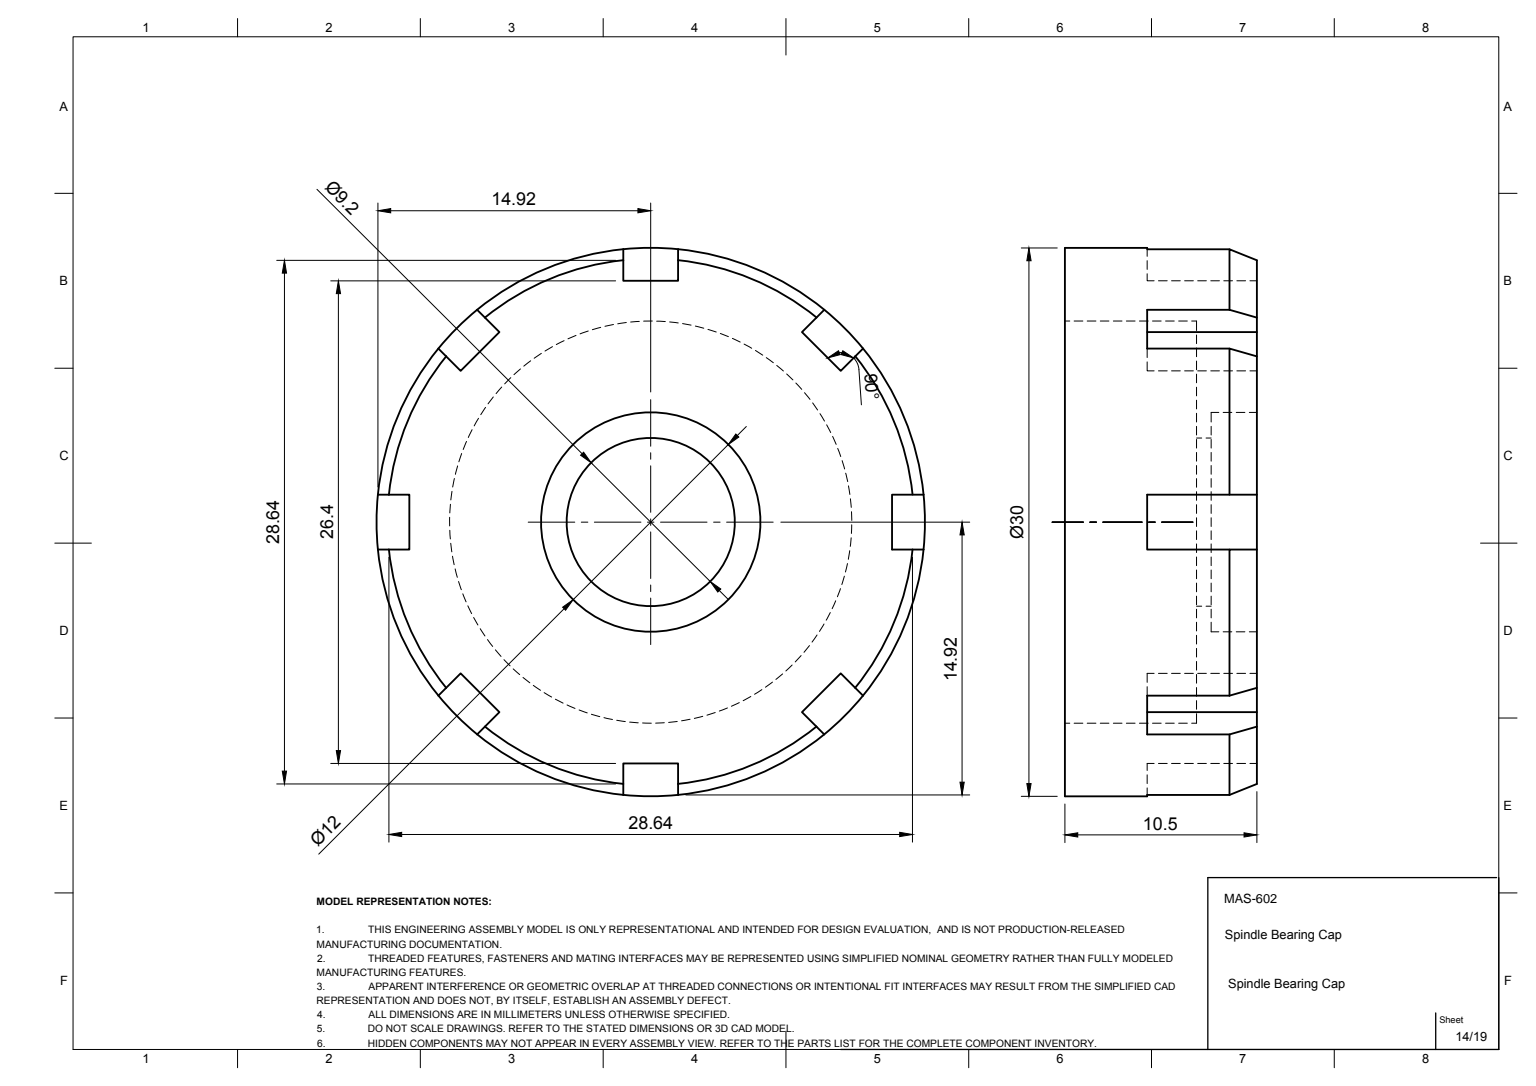
ISO-10303-21;
HEADER;
/* Generated by software containing ST-Developer
 * from STEP Tools, Inc. (www.steptools.com) 
 */

FILE_DESCRIPTION(
/* description */ (''),
/* implementation_level */ '2;1');

FILE_NAME(
/* name */ 'Spindle Bearing Cap.step',
/* time_stamp */ '2026-10-15T14:42:47-07:00',
/* author */ (''),
/* organization */ (''),
/* preprocessor_version */ 'ST-DEVELOPER v20.2',
/* originating_system */ 'Autodesk Translation Framework v15.15.0.0',
/* authorisation */ '');

FILE_SCHEMA (('AUTOMOTIVE_DESIGN { 1 0 10303 214 3 1 1 }'));
ENDSEC;

DATA;
#10=MECHANICAL_DESIGN_GEOMETRIC_PRESENTATION_REPRESENTATION('',(#242),#85789);
#131=(
BOUNDED_CURVE()
B_SPLINE_CURVE(2,(#77398,#77399,#77400),.UNSPECIFIED.,.F.,.F.)
B_SPLINE_CURVE_WITH_KNOTS((3,3),(0.,0.161672183572005),.UNSPECIFIED.)
CURVE()
GEOMETRIC_REPRESENTATION_ITEM()
RATIONAL_B_SPLINE_CURVE((1.,1.00021050527521,1.))
REPRESENTATION_ITEM('')
);
#132=(
BOUNDED_CURVE()
B_SPLINE_CURVE(2,(#77406,#77407,#77408),.UNSPECIFIED.,.F.,.F.)
B_SPLINE_CURVE_WITH_KNOTS((3,3),(0.,0.161672183572005),.UNSPECIFIED.)
CURVE()
GEOMETRIC_REPRESENTATION_ITEM()
RATIONAL_B_SPLINE_CURVE((1.,1.00021050550154,1.))
REPRESENTATION_ITEM('')
);
#133=(
BOUNDED_CURVE()
B_SPLINE_CURVE(2,(#77482,#77483,#77484),.UNSPECIFIED.,.F.,.F.)
B_SPLINE_CURVE_WITH_KNOTS((3,3),(0.,0.161672183572003),.UNSPECIFIED.)
CURVE()
GEOMETRIC_REPRESENTATION_ITEM()
RATIONAL_B_SPLINE_CURVE((1.,1.00021050513902,1.))
REPRESENTATION_ITEM('')
);
#134=(
BOUNDED_CURVE()
B_SPLINE_CURVE(2,(#77487,#77488,#77489),.UNSPECIFIED.,.F.,.F.)
B_SPLINE_CURVE_WITH_KNOTS((3,3),(0.,0.161672183572005),.UNSPECIFIED.)
CURVE()
GEOMETRIC_REPRESENTATION_ITEM()
RATIONAL_B_SPLINE_CURVE((1.,1.00021050510688,1.))
REPRESENTATION_ITEM('')
);
#135=(
BOUNDED_CURVE()
B_SPLINE_CURVE(2,(#77498,#77499,#77500),.UNSPECIFIED.,.F.,.F.)
B_SPLINE_CURVE_WITH_KNOTS((3,3),(0.,0.161672183572005),.UNSPECIFIED.)
CURVE()
GEOMETRIC_REPRESENTATION_ITEM()
RATIONAL_B_SPLINE_CURVE((1.,1.00021050528206,1.))
REPRESENTATION_ITEM('')
);
#136=(
BOUNDED_CURVE()
B_SPLINE_CURVE(2,(#77513,#77514,#77515),.UNSPECIFIED.,.F.,.F.)
B_SPLINE_CURVE_WITH_KNOTS((3,3),(0.,0.161672183572005),.UNSPECIFIED.)
CURVE()
GEOMETRIC_REPRESENTATION_ITEM()
RATIONAL_B_SPLINE_CURVE((1.,1.00021050523753,1.))
REPRESENTATION_ITEM('')
);
#137=(
BOUNDED_CURVE()
B_SPLINE_CURVE(2,(#77524,#77525,#77526),.UNSPECIFIED.,.F.,.F.)
B_SPLINE_CURVE_WITH_KNOTS((3,3),(0.,0.161672183572005),.UNSPECIFIED.)
CURVE()
GEOMETRIC_REPRESENTATION_ITEM()
RATIONAL_B_SPLINE_CURVE((1.,1.00021050533942,1.))
REPRESENTATION_ITEM('')
);
#138=(
BOUNDED_CURVE()
B_SPLINE_CURVE(2,(#77539,#77540,#77541),.UNSPECIFIED.,.F.,.F.)
B_SPLINE_CURVE_WITH_KNOTS((3,3),(0.,0.161672183572005),.UNSPECIFIED.)
CURVE()
GEOMETRIC_REPRESENTATION_ITEM()
RATIONAL_B_SPLINE_CURVE((1.,1.00021050540546,1.))
REPRESENTATION_ITEM('')
);
#139=(
BOUNDED_CURVE()
B_SPLINE_CURVE(2,(#77550,#77551,#77552),.UNSPECIFIED.,.F.,.F.)
B_SPLINE_CURVE_WITH_KNOTS((3,3),(0.,0.161672183572005),.UNSPECIFIED.)
CURVE()
GEOMETRIC_REPRESENTATION_ITEM()
RATIONAL_B_SPLINE_CURVE((1.,1.00021050533233,1.))
REPRESENTATION_ITEM('')
);
#140=(
BOUNDED_CURVE()
B_SPLINE_CURVE(2,(#77567,#77568,#77569),.UNSPECIFIED.,.F.,.F.)
B_SPLINE_CURVE_WITH_KNOTS((3,3),(0.,0.161672183572005),.UNSPECIFIED.)
CURVE()
GEOMETRIC_REPRESENTATION_ITEM()
RATIONAL_B_SPLINE_CURVE((1.,1.00021050531619,1.))
REPRESENTATION_ITEM('')
);
#141=(
BOUNDED_CURVE()
B_SPLINE_CURVE(2,(#77578,#77579,#77580),.UNSPECIFIED.,.F.,.F.)
B_SPLINE_CURVE_WITH_KNOTS((3,3),(0.,0.161672183572005),.UNSPECIFIED.)
CURVE()
GEOMETRIC_REPRESENTATION_ITEM()
RATIONAL_B_SPLINE_CURVE((1.,1.00021050600963,1.))
REPRESENTATION_ITEM('')
);
#142=(
BOUNDED_CURVE()
B_SPLINE_CURVE(2,(#77593,#77594,#77595),.UNSPECIFIED.,.F.,.F.)
B_SPLINE_CURVE_WITH_KNOTS((3,3),(0.,0.161672183572005),.UNSPECIFIED.)
CURVE()
GEOMETRIC_REPRESENTATION_ITEM()
RATIONAL_B_SPLINE_CURVE((1.,1.00021050495933,1.))
REPRESENTATION_ITEM('')
);
#143=(
BOUNDED_CURVE()
B_SPLINE_CURVE(2,(#77604,#77605,#77606),.UNSPECIFIED.,.F.,.F.)
B_SPLINE_CURVE_WITH_KNOTS((3,3),(0.,0.161672183572005),.UNSPECIFIED.)
CURVE()
GEOMETRIC_REPRESENTATION_ITEM()
RATIONAL_B_SPLINE_CURVE((1.,1.00021050494585,1.))
REPRESENTATION_ITEM('')
);
#144=(
BOUNDED_CURVE()
B_SPLINE_CURVE(2,(#77619,#77620,#77621),.UNSPECIFIED.,.F.,.F.)
B_SPLINE_CURVE_WITH_KNOTS((3,3),(0.,0.161672183572003),.UNSPECIFIED.)
CURVE()
GEOMETRIC_REPRESENTATION_ITEM()
RATIONAL_B_SPLINE_CURVE((1.,1.00021050534925,1.))
REPRESENTATION_ITEM('')
);
#145=(
BOUNDED_CURVE()
B_SPLINE_CURVE(2,(#77631,#77632,#77633),.UNSPECIFIED.,.F.,.F.)
B_SPLINE_CURVE_WITH_KNOTS((3,3),(0.,0.161672183572003),.UNSPECIFIED.)
CURVE()
GEOMETRIC_REPRESENTATION_ITEM()
RATIONAL_B_SPLINE_CURVE((1.,1.00021050497678,1.))
REPRESENTATION_ITEM('')
);
#146=(
BOUNDED_CURVE()
B_SPLINE_CURVE(2,(#77645,#77646,#77647),.UNSPECIFIED.,.F.,.F.)
B_SPLINE_CURVE_WITH_KNOTS((3,3),(0.,0.161672183572003),.UNSPECIFIED.)
CURVE()
GEOMETRIC_REPRESENTATION_ITEM()
RATIONAL_B_SPLINE_CURVE((1.,1.00021050515309,1.))
REPRESENTATION_ITEM('')
);
#169=CONICAL_SURFACE('',#10614,1.47,0.380506377112364);
#170=CONICAL_SURFACE('',#10616,1.47,0.380506377112364);
#171=CONICAL_SURFACE('',#10623,1.47,0.380506377112364);
#172=CONICAL_SURFACE('',#10630,1.47,0.380506377112364);
#173=CONICAL_SURFACE('',#10638,1.47,0.380506377112364);
#174=CONICAL_SURFACE('',#10645,1.47,0.380506377112364);
#175=CONICAL_SURFACE('',#10652,1.47,0.380506377112364);
#176=CONICAL_SURFACE('',#10659,1.47,0.380506377112364);
#206=SHAPE_REPRESENTATION_RELATIONSHIP('SRR','None',#85871,#224);
#224=ADVANCED_BREP_SHAPE_REPRESENTATION('',(#260),#85779);
#242=STYLED_ITEM('',(#85970),#260);
#260=MANIFOLD_SOLID_BREP('Body1',#9889);
#455=FACE_BOUND('',#3306,.T.);
#456=FACE_BOUND('',#3345,.T.);
#457=FACE_BOUND('',#3348,.T.);
#458=FACE_BOUND('',#3352,.T.);
#1118=PLANE('',#10599);
#1119=PLANE('',#10600);
#1120=PLANE('',#10601);
#1121=PLANE('',#10602);
#1122=PLANE('',#10604);
#1123=PLANE('',#10618);
#1124=PLANE('',#10619);
#1125=PLANE('',#10620);
#1126=PLANE('',#10621);
#1127=PLANE('',#10625);
#1128=PLANE('',#10626);
#1129=PLANE('',#10627);
#1130=PLANE('',#10628);
#1131=PLANE('',#10632);
#1132=PLANE('',#10633);
#1133=PLANE('',#10634);
#1134=PLANE('',#10635);
#1135=PLANE('',#10640);
#1136=PLANE('',#10641);
#1137=PLANE('',#10642);
#1138=PLANE('',#10643);
#1139=PLANE('',#10647);
#1140=PLANE('',#10648);
#1141=PLANE('',#10649);
#1142=PLANE('',#10650);
#1143=PLANE('',#10654);
#1144=PLANE('',#10655);
#1145=PLANE('',#10656);
#1146=PLANE('',#10657);
#1147=PLANE('',#10661);
#1148=PLANE('',#10662);
#1149=PLANE('',#10663);
#1150=PLANE('',#10664);
#1151=PLANE('',#10669);
#1152=PLANE('',#10673);
#1153=PLANE('',#10678);
#1539=LINE('',#77391,#2075);
#1540=LINE('',#77393,#2076);
#1541=LINE('',#77395,#2077);
#1542=LINE('',#77397,#2078);
#1543=LINE('',#77404,#2079);
#1544=LINE('',#77410,#2080);
#1545=LINE('',#77412,#2081);
#1546=LINE('',#77413,#2082);
#1547=LINE('',#77415,#2083);
#1548=LINE('',#77416,#2084);
#1549=LINE('',#77423,#2085);
#1550=LINE('',#77425,#2086);
#1551=LINE('',#77427,#2087);
#1552=LINE('',#77431,#2088);
#1553=LINE('',#77433,#2089);
#1554=LINE('',#77435,#2090);
#1555=LINE('',#77439,#2091);
#1556=LINE('',#77441,#2092);
#1557=LINE('',#77443,#2093);
#1558=LINE('',#77447,#2094);
#1559=LINE('',#77449,#2095);
#1560=LINE('',#77451,#2096);
#1561=LINE('',#77455,#2097);
#1562=LINE('',#77457,#2098);
#1563=LINE('',#77459,#2099);
#1564=LINE('',#77463,#2100);
#1565=LINE('',#77465,#2101);
#1566=LINE('',#77467,#2102);
#1567=LINE('',#77471,#2103);
#1568=LINE('',#77473,#2104);
#1569=LINE('',#77475,#2105);
#1570=LINE('',#77494,#2106);
#1571=LINE('',#77496,#2107);
#1572=LINE('',#77497,#2108);
#1573=LINE('',#77503,#2109);
#1574=LINE('',#77505,#2110);
#1575=LINE('',#77506,#2111);
#1576=LINE('',#77508,#2112);
#1577=LINE('',#77520,#2113);
#1578=LINE('',#77522,#2114);
#1579=LINE('',#77523,#2115);
#1580=LINE('',#77529,#2116);
#1581=LINE('',#77531,#2117);
#1582=LINE('',#77532,#2118);
#1583=LINE('',#77534,#2119);
#1584=LINE('',#77546,#2120);
#1585=LINE('',#77548,#2121);
#1586=LINE('',#77549,#2122);
#1587=LINE('',#77555,#2123);
#1588=LINE('',#77557,#2124);
#1589=LINE('',#77558,#2125);
#1590=LINE('',#77560,#2126);
#1591=LINE('',#77574,#2127);
#1592=LINE('',#77576,#2128);
#1593=LINE('',#77577,#2129);
#1594=LINE('',#77583,#2130);
#1595=LINE('',#77585,#2131);
#1596=LINE('',#77586,#2132);
#1597=LINE('',#77588,#2133);
#1598=LINE('',#77600,#2134);
#1599=LINE('',#77602,#2135);
#1600=LINE('',#77603,#2136);
#1601=LINE('',#77609,#2137);
#1602=LINE('',#77611,#2138);
#1603=LINE('',#77612,#2139);
#1604=LINE('',#77614,#2140);
#1605=LINE('',#77625,#2141);
#1606=LINE('',#77627,#2142);
#1607=LINE('',#77628,#2143);
#1608=LINE('',#77635,#2144);
#1609=LINE('',#77637,#2145);
#1610=LINE('',#77638,#2146);
#1611=LINE('',#77640,#2147);
#1612=LINE('',#77651,#2148);
#1613=LINE('',#77653,#2149);
#1614=LINE('',#77654,#2150);
#1615=LINE('',#77657,#2151);
#1616=LINE('',#77659,#2152);
#1617=LINE('',#77660,#2153);
#1618=LINE('',#77662,#2154);
#1619=LINE('',#77669,#2155);
#1620=LINE('',#77676,#2156);
#1621=LINE('',#77682,#2157);
#1622=LINE('',#77686,#2158);
#2075=VECTOR('',#12303,1.);
#2076=VECTOR('',#12304,1.);
#2077=VECTOR('',#12305,1.);
#2078=VECTOR('',#12306,1.);
#2079=VECTOR('',#12309,1.);
#2080=VECTOR('',#12310,1.);
#2081=VECTOR('',#12311,1.);
#2082=VECTOR('',#12312,1.);
#2083=VECTOR('',#12315,1.);
#2084=VECTOR('',#12316,1.);
#2085=VECTOR('',#12325,1.);
#2086=VECTOR('',#12326,1.);
#2087=VECTOR('',#12327,1.);
#2088=VECTOR('',#12330,1.);
#2089=VECTOR('',#12331,1.);
#2090=VECTOR('',#12332,1.);
#2091=VECTOR('',#12335,1.);
#2092=VECTOR('',#12336,1.);
#2093=VECTOR('',#12337,1.);
#2094=VECTOR('',#12340,1.);
#2095=VECTOR('',#12341,1.);
#2096=VECTOR('',#12342,1.);
#2097=VECTOR('',#12345,1.);
#2098=VECTOR('',#12346,1.);
#2099=VECTOR('',#12347,1.);
#2100=VECTOR('',#12350,1.);
#2101=VECTOR('',#12351,1.);
#2102=VECTOR('',#12352,1.);
#2103=VECTOR('',#12355,1.);
#2104=VECTOR('',#12356,1.);
#2105=VECTOR('',#12357,1.);
#2106=VECTOR('',#12372,1.);
#2107=VECTOR('',#12373,1.);
#2108=VECTOR('',#12374,1.);
#2109=VECTOR('',#12377,1.);
#2110=VECTOR('',#12378,1.);
#2111=VECTOR('',#12379,1.);
#2112=VECTOR('',#12382,1.);
#2113=VECTOR('',#12393,1.);
#2114=VECTOR('',#12394,1.);
#2115=VECTOR('',#12395,1.);
#2116=VECTOR('',#12398,1.);
#2117=VECTOR('',#12399,1.);
#2118=VECTOR('',#12400,1.);
#2119=VECTOR('',#12403,1.);
#2120=VECTOR('',#12414,1.);
#2121=VECTOR('',#12415,1.);
#2122=VECTOR('',#12416,1.);
#2123=VECTOR('',#12419,1.);
#2124=VECTOR('',#12420,1.);
#2125=VECTOR('',#12421,1.);
#2126=VECTOR('',#12424,1.);
#2127=VECTOR('',#12437,1.);
#2128=VECTOR('',#12438,1.);
#2129=VECTOR('',#12439,1.);
#2130=VECTOR('',#12442,1.);
#2131=VECTOR('',#12443,1.);
#2132=VECTOR('',#12444,1.);
#2133=VECTOR('',#12447,1.);
#2134=VECTOR('',#12458,1.);
#2135=VECTOR('',#12459,1.);
#2136=VECTOR('',#12460,1.);
#2137=VECTOR('',#12463,1.);
#2138=VECTOR('',#12464,1.);
#2139=VECTOR('',#12465,1.);
#2140=VECTOR('',#12468,1.);
#2141=VECTOR('',#12479,1.);
#2142=VECTOR('',#12480,1.);
#2143=VECTOR('',#12481,1.);
#2144=VECTOR('',#12484,1.);
#2145=VECTOR('',#12485,1.);
#2146=VECTOR('',#12486,1.);
#2147=VECTOR('',#12489,1.);
#2148=VECTOR('',#12500,1.);
#2149=VECTOR('',#12501,1.);
#2150=VECTOR('',#12502,1.);
#2151=VECTOR('',#12505,1.);
#2152=VECTOR('',#12506,1.);
#2153=VECTOR('',#12507,1.);
#2154=VECTOR('',#12510,1.);
#2155=VECTOR('',#12519,1.1);
#2156=VECTOR('',#12528,0.46);
#2157=VECTOR('',#12537,1.5);
#2158=VECTOR('',#12542,0.6);
#2344=CYLINDRICAL_SURFACE('',#10666,1.1);
#2345=CYLINDRICAL_SURFACE('',#10671,0.46);
#2346=CYLINDRICAL_SURFACE('',#10675,1.5);
#2347=CYLINDRICAL_SURFACE('',#10676,0.6);
#2731=FACE_OUTER_BOUND('',#3301,.T.);
#2732=FACE_OUTER_BOUND('',#3302,.T.);
#2733=FACE_OUTER_BOUND('',#3303,.T.);
#2734=FACE_OUTER_BOUND('',#3304,.T.);
#2735=FACE_OUTER_BOUND('',#3305,.T.);
#2736=FACE_OUTER_BOUND('',#3307,.T.);
#2737=FACE_OUTER_BOUND('',#3308,.T.);
#2738=FACE_OUTER_BOUND('',#3309,.T.);
#2739=FACE_OUTER_BOUND('',#3310,.T.);
#2740=FACE_OUTER_BOUND('',#3311,.T.);
#2741=FACE_OUTER_BOUND('',#3312,.T.);
#2742=FACE_OUTER_BOUND('',#3313,.T.);
#2743=FACE_OUTER_BOUND('',#3314,.T.);
#2744=FACE_OUTER_BOUND('',#3315,.T.);
#2745=FACE_OUTER_BOUND('',#3316,.T.);
#2746=FACE_OUTER_BOUND('',#3317,.T.);
#2747=FACE_OUTER_BOUND('',#3318,.T.);
#2748=FACE_OUTER_BOUND('',#3319,.T.);
#2749=FACE_OUTER_BOUND('',#3320,.T.);
#2750=FACE_OUTER_BOUND('',#3321,.T.);
#2751=FACE_OUTER_BOUND('',#3322,.T.);
#2752=FACE_OUTER_BOUND('',#3323,.T.);
#2753=FACE_OUTER_BOUND('',#3324,.T.);
#2754=FACE_OUTER_BOUND('',#3325,.T.);
#2755=FACE_OUTER_BOUND('',#3326,.T.);
#2756=FACE_OUTER_BOUND('',#3327,.T.);
#2757=FACE_OUTER_BOUND('',#3328,.T.);
#2758=FACE_OUTER_BOUND('',#3329,.T.);
#2759=FACE_OUTER_BOUND('',#3330,.T.);
#2760=FACE_OUTER_BOUND('',#3331,.T.);
#2761=FACE_OUTER_BOUND('',#3332,.T.);
#2762=FACE_OUTER_BOUND('',#3333,.T.);
#2763=FACE_OUTER_BOUND('',#3334,.T.);
#2764=FACE_OUTER_BOUND('',#3335,.T.);
#2765=FACE_OUTER_BOUND('',#3336,.T.);
#2766=FACE_OUTER_BOUND('',#3337,.T.);
#2767=FACE_OUTER_BOUND('',#3338,.T.);
#2768=FACE_OUTER_BOUND('',#3339,.T.);
#2769=FACE_OUTER_BOUND('',#3340,.T.);
#2770=FACE_OUTER_BOUND('',#3341,.T.);
#2771=FACE_OUTER_BOUND('',#3342,.T.);
#2772=FACE_OUTER_BOUND('',#3343,.T.);
#2773=FACE_OUTER_BOUND('',#3344,.T.);
#2774=FACE_OUTER_BOUND('',#3346,.T.);
#2775=FACE_OUTER_BOUND('',#3347,.T.);
#2776=FACE_OUTER_BOUND('',#3349,.T.);
#2777=FACE_OUTER_BOUND('',#3350,.T.);
#2778=FACE_OUTER_BOUND('',#3351,.T.);
#3301=EDGE_LOOP('',(#8463,#8464,#8465,#8466,#8467));
#3302=EDGE_LOOP('',(#8468,#8469,#8470,#8471,#8472));
#3303=EDGE_LOOP('',(#8473,#8474,#8475,#8476));
#3304=EDGE_LOOP('',(#8477,#8478,#8479,#8480));
#3305=EDGE_LOOP('',(#8481,#8482,#8483,#8484,#8485,#8486,#8487,#8488,#8489,
#8490,#8491,#8492,#8493,#8494,#8495,#8496,#8497,#8498,#8499,#8500,#8501,
#8502,#8503,#8504,#8505,#8506,#8507,#8508,#8509,#8510,#8511,#8512));
#3306=EDGE_LOOP('',(#8513));
#3307=EDGE_LOOP('',(#8514,#8515,#8516,#8517));
#3308=EDGE_LOOP('',(#8518,#8519,#8520,#8521));
#3309=EDGE_LOOP('',(#8522,#8523,#8524,#8525,#8526));
#3310=EDGE_LOOP('',(#8527,#8528,#8529,#8530,#8531));
#3311=EDGE_LOOP('',(#8532,#8533,#8534,#8535));
#3312=EDGE_LOOP('',(#8536,#8537,#8538,#8539));
#3313=EDGE_LOOP('',(#8540,#8541,#8542,#8543));
#3314=EDGE_LOOP('',(#8544,#8545,#8546,#8547,#8548));
#3315=EDGE_LOOP('',(#8549,#8550,#8551,#8552,#8553));
#3316=EDGE_LOOP('',(#8554,#8555,#8556,#8557));
#3317=EDGE_LOOP('',(#8558,#8559,#8560,#8561));
#3318=EDGE_LOOP('',(#8562,#8563,#8564,#8565));
#3319=EDGE_LOOP('',(#8566,#8567,#8568,#8569,#8570));
#3320=EDGE_LOOP('',(#8571,#8572,#8573,#8574,#8575));
#3321=EDGE_LOOP('',(#8576,#8577,#8578,#8579));
#3322=EDGE_LOOP('',(#8580,#8581,#8582,#8583,#8584));
#3323=EDGE_LOOP('',(#8585,#8586,#8587,#8588));
#3324=EDGE_LOOP('',(#8589,#8590,#8591,#8592,#8593));
#3325=EDGE_LOOP('',(#8594,#8595,#8596,#8597,#8598));
#3326=EDGE_LOOP('',(#8599,#8600,#8601,#8602));
#3327=EDGE_LOOP('',(#8603,#8604,#8605,#8606));
#3328=EDGE_LOOP('',(#8607,#8608,#8609,#8610));
#3329=EDGE_LOOP('',(#8611,#8612,#8613,#8614,#8615));
#3330=EDGE_LOOP('',(#8616,#8617,#8618,#8619,#8620));
#3331=EDGE_LOOP('',(#8621,#8622,#8623,#8624));
#3332=EDGE_LOOP('',(#8625,#8626,#8627,#8628));
#3333=EDGE_LOOP('',(#8629,#8630,#8631,#8632));
#3334=EDGE_LOOP('',(#8633,#8634,#8635,#8636,#8637));
#3335=EDGE_LOOP('',(#8638,#8639,#8640,#8641,#8642));
#3336=EDGE_LOOP('',(#8643,#8644,#8645,#8646));
#3337=EDGE_LOOP('',(#8647,#8648,#8649,#8650));
#3338=EDGE_LOOP('',(#8651,#8652,#8653,#8654));
#3339=EDGE_LOOP('',(#8655,#8656,#8657,#8658,#8659));
#3340=EDGE_LOOP('',(#8660,#8661,#8662,#8663,#8664));
#3341=EDGE_LOOP('',(#8665,#8666,#8667,#8668));
#3342=EDGE_LOOP('',(#8669,#8670,#8671,#8672));
#3343=EDGE_LOOP('',(#8673,#8674,#8675,#8676));
#3344=EDGE_LOOP('',(#8677));
#3345=EDGE_LOOP('',(#8678));
#3346=EDGE_LOOP('',(#8679,#8680,#8681,#8682));
#3347=EDGE_LOOP('',(#8683));
#3348=EDGE_LOOP('',(#8684));
#3349=EDGE_LOOP('',(#8685,#8686,#8687,#8688,#8689,#8690,#8691,#8692,#8693,
#8694,#8695,#8696,#8697,#8698,#8699,#8700,#8701,#8702,#8703,#8704,#8705,
#8706,#8707,#8708,#8709,#8710,#8711,#8712,#8713,#8714,#8715,#8716,#8717,
#8718,#8719,#8720));
#3350=EDGE_LOOP('',(#8721,#8722,#8723,#8724));
#3351=EDGE_LOOP('',(#8725));
#3352=EDGE_LOOP('',(#8726));
#3744=CIRCLE('',#10603,1.5);
#3745=CIRCLE('',#10605,1.44);
#3746=CIRCLE('',#10606,1.44);
#3747=CIRCLE('',#10607,1.44);
#3748=CIRCLE('',#10608,1.44);
#3749=CIRCLE('',#10609,1.44);
#3750=CIRCLE('',#10610,1.44);
#3751=CIRCLE('',#10611,1.44);
#3752=CIRCLE('',#10612,1.44);
#3753=CIRCLE('',#10613,0.6);
#3754=CIRCLE('',#10615,1.5);
#3755=CIRCLE('',#10617,1.5);
#3756=CIRCLE('',#10622,1.5);
#3757=CIRCLE('',#10624,1.5);
#3758=CIRCLE('',#10629,1.5);
#3759=CIRCLE('',#10631,1.5);
#3760=CIRCLE('',#10636,1.5);
#3761=CIRCLE('',#10637,1.5);
#3762=CIRCLE('',#10639,1.5);
#3763=CIRCLE('',#10644,1.5);
#3764=CIRCLE('',#10646,1.5);
#3765=CIRCLE('',#10651,1.5);
#3766=CIRCLE('',#10653,1.5);
#3767=CIRCLE('',#10658,1.5);
#3768=CIRCLE('',#10660,1.5);
#3769=CIRCLE('',#10665,1.5);
#3770=CIRCLE('',#10667,1.1);
#3771=CIRCLE('',#10668,1.1);
#3772=CIRCLE('',#10670,0.46);
#3773=CIRCLE('',#10672,0.46);
#3774=CIRCLE('',#10674,1.5);
#3775=CIRCLE('',#10677,0.6);
#4619=VERTEX_POINT('',#77389);
#4620=VERTEX_POINT('',#77390);
#4621=VERTEX_POINT('',#77392);
#4622=VERTEX_POINT('',#77394);
#4623=VERTEX_POINT('',#77396);
#4624=VERTEX_POINT('',#77402);
#4625=VERTEX_POINT('',#77403);
#4626=VERTEX_POINT('',#77405);
#4627=VERTEX_POINT('',#77409);
#4628=VERTEX_POINT('',#77411);
#4629=VERTEX_POINT('',#77420);
#4630=VERTEX_POINT('',#77422);
#4631=VERTEX_POINT('',#77424);
#4632=VERTEX_POINT('',#77426);
#4633=VERTEX_POINT('',#77428);
#4634=VERTEX_POINT('',#77430);
#4635=VERTEX_POINT('',#77432);
#4636=VERTEX_POINT('',#77434);
#4637=VERTEX_POINT('',#77436);
#4638=VERTEX_POINT('',#77438);
#4639=VERTEX_POINT('',#77440);
#4640=VERTEX_POINT('',#77442);
#4641=VERTEX_POINT('',#77444);
#4642=VERTEX_POINT('',#77446);
#4643=VERTEX_POINT('',#77448);
#4644=VERTEX_POINT('',#77450);
#4645=VERTEX_POINT('',#77452);
#4646=VERTEX_POINT('',#77454);
#4647=VERTEX_POINT('',#77456);
#4648=VERTEX_POINT('',#77458);
#4649=VERTEX_POINT('',#77460);
#4650=VERTEX_POINT('',#77462);
#4651=VERTEX_POINT('',#77464);
#4652=VERTEX_POINT('',#77466);
#4653=VERTEX_POINT('',#77468);
#4654=VERTEX_POINT('',#77470);
#4655=VERTEX_POINT('',#77472);
#4656=VERTEX_POINT('',#77474);
#4657=VERTEX_POINT('',#77477);
#4658=VERTEX_POINT('',#77480);
#4659=VERTEX_POINT('',#77486);
#4660=VERTEX_POINT('',#77492);
#4661=VERTEX_POINT('',#77493);
#4662=VERTEX_POINT('',#77495);
#4663=VERTEX_POINT('',#77502);
#4664=VERTEX_POINT('',#77504);
#4665=VERTEX_POINT('',#77512);
#4666=VERTEX_POINT('',#77518);
#4667=VERTEX_POINT('',#77519);
#4668=VERTEX_POINT('',#77521);
#4669=VERTEX_POINT('',#77528);
#4670=VERTEX_POINT('',#77530);
#4671=VERTEX_POINT('',#77538);
#4672=VERTEX_POINT('',#77544);
#4673=VERTEX_POINT('',#77545);
#4674=VERTEX_POINT('',#77547);
#4675=VERTEX_POINT('',#77554);
#4676=VERTEX_POINT('',#77556);
#4677=VERTEX_POINT('',#77562);
#4678=VERTEX_POINT('',#77566);
#4679=VERTEX_POINT('',#77572);
#4680=VERTEX_POINT('',#77573);
#4681=VERTEX_POINT('',#77575);
#4682=VERTEX_POINT('',#77582);
#4683=VERTEX_POINT('',#77584);
#4684=VERTEX_POINT('',#77592);
#4685=VERTEX_POINT('',#77598);
#4686=VERTEX_POINT('',#77599);
#4687=VERTEX_POINT('',#77601);
#4688=VERTEX_POINT('',#77608);
#4689=VERTEX_POINT('',#77610);
#4690=VERTEX_POINT('',#77618);
#4691=VERTEX_POINT('',#77624);
#4692=VERTEX_POINT('',#77626);
#4693=VERTEX_POINT('',#77630);
#4694=VERTEX_POINT('',#77634);
#4695=VERTEX_POINT('',#77636);
#4696=VERTEX_POINT('',#77644);
#4697=VERTEX_POINT('',#77650);
#4698=VERTEX_POINT('',#77652);
#4699=VERTEX_POINT('',#77656);
#4700=VERTEX_POINT('',#77658);
#4701=VERTEX_POINT('',#77666);
#4702=VERTEX_POINT('',#77668);
#4703=VERTEX_POINT('',#77672);
#4704=VERTEX_POINT('',#77675);
#4705=VERTEX_POINT('',#77679);
#4706=VERTEX_POINT('',#77684);
#5959=EDGE_CURVE('',#4619,#4620,#1539,.T.);
#5960=EDGE_CURVE('',#4619,#4621,#1540,.T.);
#5961=EDGE_CURVE('',#4622,#4621,#1541,.T.);
#5962=EDGE_CURVE('',#4623,#4622,#1542,.T.);
#5963=EDGE_CURVE('',#4620,#4623,#131,.T.);
#5964=EDGE_CURVE('',#4624,#4625,#1543,.T.);
#5965=EDGE_CURVE('',#4626,#4624,#132,.T.);
#5966=EDGE_CURVE('',#4627,#4626,#1544,.T.);
#5967=EDGE_CURVE('',#4627,#4628,#1545,.T.);
#5968=EDGE_CURVE('',#4628,#4625,#1546,.T.);
#5969=EDGE_CURVE('',#4622,#4627,#1547,.T.);
#5970=EDGE_CURVE('',#4621,#4628,#1548,.T.);
#5971=EDGE_CURVE('',#4625,#4619,#3744,.T.);
#5972=EDGE_CURVE('',#4626,#4629,#3745,.T.);
#5973=EDGE_CURVE('',#4629,#4630,#1549,.T.);
#5974=EDGE_CURVE('',#4630,#4631,#1550,.T.);
#5975=EDGE_CURVE('',#4631,#4632,#1551,.T.);
#5976=EDGE_CURVE('',#4632,#4633,#3746,.T.);
#5977=EDGE_CURVE('',#4633,#4634,#1552,.T.);
#5978=EDGE_CURVE('',#4634,#4635,#1553,.T.);
#5979=EDGE_CURVE('',#4635,#4636,#1554,.T.);
#5980=EDGE_CURVE('',#4636,#4637,#3747,.T.);
#5981=EDGE_CURVE('',#4637,#4638,#1555,.T.);
#5982=EDGE_CURVE('',#4638,#4639,#1556,.T.);
#5983=EDGE_CURVE('',#4639,#4640,#1557,.T.);
#5984=EDGE_CURVE('',#4640,#4641,#3748,.T.);
#5985=EDGE_CURVE('',#4641,#4642,#1558,.T.);
#5986=EDGE_CURVE('',#4642,#4643,#1559,.T.);
#5987=EDGE_CURVE('',#4643,#4644,#1560,.T.);
#5988=EDGE_CURVE('',#4644,#4645,#3749,.T.);
#5989=EDGE_CURVE('',#4645,#4646,#1561,.T.);
#5990=EDGE_CURVE('',#4646,#4647,#1562,.T.);
#5991=EDGE_CURVE('',#4647,#4648,#1563,.T.);
#5992=EDGE_CURVE('',#4648,#4649,#3750,.T.);
#5993=EDGE_CURVE('',#4649,#4650,#1564,.T.);
#5994=EDGE_CURVE('',#4650,#4651,#1565,.T.);
#5995=EDGE_CURVE('',#4651,#4652,#1566,.T.);
#5996=EDGE_CURVE('',#4652,#4653,#3751,.T.);
#5997=EDGE_CURVE('',#4653,#4654,#1567,.T.);
#5998=EDGE_CURVE('',#4654,#4655,#1568,.T.);
#5999=EDGE_CURVE('',#4655,#4656,#1569,.T.);
#6000=EDGE_CURVE('',#4656,#4623,#3752,.T.);
#6001=EDGE_CURVE('',#4657,#4657,#3753,.T.);
#6002=EDGE_CURVE('',#4624,#4658,#3754,.T.);
#6003=EDGE_CURVE('',#4658,#4629,#133,.T.);
#6004=EDGE_CURVE('',#4656,#4659,#134,.T.);
#6005=EDGE_CURVE('',#4659,#4620,#3755,.T.);
#6006=EDGE_CURVE('',#4660,#4661,#1570,.T.);
#6007=EDGE_CURVE('',#4660,#4662,#1571,.T.);
#6008=EDGE_CURVE('',#4654,#4662,#1572,.T.);
#6009=EDGE_CURVE('',#4661,#4653,#135,.T.);
#6010=EDGE_CURVE('',#4659,#4663,#1573,.T.);
#6011=EDGE_CURVE('',#4655,#4664,#1574,.T.);
#6012=EDGE_CURVE('',#4664,#4663,#1575,.T.);
#6013=EDGE_CURVE('',#4662,#4664,#1576,.T.);
#6014=EDGE_CURVE('',#4663,#4660,#3756,.T.);
#6015=EDGE_CURVE('',#4652,#4665,#136,.T.);
#6016=EDGE_CURVE('',#4665,#4661,#3757,.T.);
#6017=EDGE_CURVE('',#4666,#4667,#1577,.T.);
#6018=EDGE_CURVE('',#4666,#4668,#1578,.T.);
#6019=EDGE_CURVE('',#4650,#4668,#1579,.T.);
#6020=EDGE_CURVE('',#4667,#4649,#137,.T.);
#6021=EDGE_CURVE('',#4665,#4669,#1580,.T.);
#6022=EDGE_CURVE('',#4651,#4670,#1581,.T.);
#6023=EDGE_CURVE('',#4670,#4669,#1582,.T.);
#6024=EDGE_CURVE('',#4668,#4670,#1583,.T.);
#6025=EDGE_CURVE('',#4669,#4666,#3758,.T.);
#6026=EDGE_CURVE('',#4648,#4671,#138,.T.);
#6027=EDGE_CURVE('',#4671,#4667,#3759,.T.);
#6028=EDGE_CURVE('',#4672,#4673,#1584,.T.);
#6029=EDGE_CURVE('',#4672,#4674,#1585,.T.);
#6030=EDGE_CURVE('',#4646,#4674,#1586,.T.);
#6031=EDGE_CURVE('',#4673,#4645,#139,.T.);
#6032=EDGE_CURVE('',#4671,#4675,#1587,.T.);
#6033=EDGE_CURVE('',#4647,#4676,#1588,.T.);
#6034=EDGE_CURVE('',#4676,#4675,#1589,.T.);
#6035=EDGE_CURVE('',#4674,#4676,#1590,.T.);
#6036=EDGE_CURVE('',#4675,#4677,#3760,.T.);
#6037=EDGE_CURVE('',#4677,#4672,#3761,.T.);
#6038=EDGE_CURVE('',#4644,#4678,#140,.T.);
#6039=EDGE_CURVE('',#4678,#4673,#3762,.T.);
#6040=EDGE_CURVE('',#4679,#4680,#1591,.T.);
#6041=EDGE_CURVE('',#4679,#4681,#1592,.T.);
#6042=EDGE_CURVE('',#4642,#4681,#1593,.T.);
#6043=EDGE_CURVE('',#4680,#4641,#141,.T.);
#6044=EDGE_CURVE('',#4678,#4682,#1594,.T.);
#6045=EDGE_CURVE('',#4643,#4683,#1595,.T.);
#6046=EDGE_CURVE('',#4683,#4682,#1596,.T.);
#6047=EDGE_CURVE('',#4681,#4683,#1597,.T.);
#6048=EDGE_CURVE('',#4682,#4679,#3763,.T.);
#6049=EDGE_CURVE('',#4640,#4684,#142,.T.);
#6050=EDGE_CURVE('',#4684,#4680,#3764,.T.);
#6051=EDGE_CURVE('',#4685,#4686,#1598,.T.);
#6052=EDGE_CURVE('',#4685,#4687,#1599,.T.);
#6053=EDGE_CURVE('',#4638,#4687,#1600,.T.);
#6054=EDGE_CURVE('',#4686,#4637,#143,.T.);
#6055=EDGE_CURVE('',#4684,#4688,#1601,.T.);
#6056=EDGE_CURVE('',#4639,#4689,#1602,.T.);
#6057=EDGE_CURVE('',#4689,#4688,#1603,.T.);
#6058=EDGE_CURVE('',#4687,#4689,#1604,.T.);
#6059=EDGE_CURVE('',#4688,#4685,#3765,.T.);
#6060=EDGE_CURVE('',#4636,#4690,#144,.T.);
#6061=EDGE_CURVE('',#4690,#4686,#3766,.T.);
#6062=EDGE_CURVE('',#4635,#4691,#1605,.T.);
#6063=EDGE_CURVE('',#4691,#4692,#1606,.T.);
#6064=EDGE_CURVE('',#4690,#4692,#1607,.T.);
#6065=EDGE_CURVE('',#4693,#4633,#145,.T.);
#6066=EDGE_CURVE('',#4694,#4693,#1608,.T.);
#6067=EDGE_CURVE('',#4694,#4695,#1609,.T.);
#6068=EDGE_CURVE('',#4634,#4695,#1610,.T.);
#6069=EDGE_CURVE('',#4695,#4691,#1611,.T.);
#6070=EDGE_CURVE('',#4692,#4694,#3767,.T.);
#6071=EDGE_CURVE('',#4632,#4696,#146,.T.);
#6072=EDGE_CURVE('',#4696,#4693,#3768,.T.);
#6073=EDGE_CURVE('',#4631,#4697,#1612,.T.);
#6074=EDGE_CURVE('',#4697,#4698,#1613,.T.);
#6075=EDGE_CURVE('',#4696,#4698,#1614,.T.);
#6076=EDGE_CURVE('',#4699,#4658,#1615,.T.);
#6077=EDGE_CURVE('',#4699,#4700,#1616,.T.);
#6078=EDGE_CURVE('',#4630,#4700,#1617,.T.);
#6079=EDGE_CURVE('',#4700,#4697,#1618,.T.);
#6080=EDGE_CURVE('',#4698,#4699,#3769,.T.);
#6081=EDGE_CURVE('',#4701,#4701,#3770,.T.);
#6082=EDGE_CURVE('',#4701,#4702,#1619,.T.);
#6083=EDGE_CURVE('',#4702,#4702,#3771,.T.);
#6084=EDGE_CURVE('',#4703,#4703,#3772,.T.);
#6085=EDGE_CURVE('',#4703,#4704,#1620,.T.);
#6086=EDGE_CURVE('',#4704,#4704,#3773,.T.);
#6087=EDGE_CURVE('',#4705,#4705,#3774,.T.);
#6088=EDGE_CURVE('',#4677,#4705,#1621,.T.);
#6089=EDGE_CURVE('',#4706,#4706,#3775,.T.);
#6090=EDGE_CURVE('',#4706,#4657,#1622,.T.);
#8463=ORIENTED_EDGE('',*,*,#5959,.F.);
#8464=ORIENTED_EDGE('',*,*,#5960,.T.);
#8465=ORIENTED_EDGE('',*,*,#5961,.F.);
#8466=ORIENTED_EDGE('',*,*,#5962,.F.);
#8467=ORIENTED_EDGE('',*,*,#5963,.F.);
#8468=ORIENTED_EDGE('',*,*,#5964,.F.);
#8469=ORIENTED_EDGE('',*,*,#5965,.F.);
#8470=ORIENTED_EDGE('',*,*,#5966,.F.);
#8471=ORIENTED_EDGE('',*,*,#5967,.T.);
#8472=ORIENTED_EDGE('',*,*,#5968,.T.);
#8473=ORIENTED_EDGE('',*,*,#5969,.F.);
#8474=ORIENTED_EDGE('',*,*,#5961,.T.);
#8475=ORIENTED_EDGE('',*,*,#5970,.T.);
#8476=ORIENTED_EDGE('',*,*,#5967,.F.);
#8477=ORIENTED_EDGE('',*,*,#5971,.F.);
#8478=ORIENTED_EDGE('',*,*,#5968,.F.);
#8479=ORIENTED_EDGE('',*,*,#5970,.F.);
#8480=ORIENTED_EDGE('',*,*,#5960,.F.);
#8481=ORIENTED_EDGE('',*,*,#5962,.T.);
#8482=ORIENTED_EDGE('',*,*,#5969,.T.);
#8483=ORIENTED_EDGE('',*,*,#5966,.T.);
#8484=ORIENTED_EDGE('',*,*,#5972,.T.);
#8485=ORIENTED_EDGE('',*,*,#5973,.T.);
#8486=ORIENTED_EDGE('',*,*,#5974,.T.);
#8487=ORIENTED_EDGE('',*,*,#5975,.T.);
#8488=ORIENTED_EDGE('',*,*,#5976,.T.);
#8489=ORIENTED_EDGE('',*,*,#5977,.T.);
#8490=ORIENTED_EDGE('',*,*,#5978,.T.);
#8491=ORIENTED_EDGE('',*,*,#5979,.T.);
#8492=ORIENTED_EDGE('',*,*,#5980,.T.);
#8493=ORIENTED_EDGE('',*,*,#5981,.T.);
#8494=ORIENTED_EDGE('',*,*,#5982,.T.);
#8495=ORIENTED_EDGE('',*,*,#5983,.T.);
#8496=ORIENTED_EDGE('',*,*,#5984,.T.);
#8497=ORIENTED_EDGE('',*,*,#5985,.T.);
#8498=ORIENTED_EDGE('',*,*,#5986,.T.);
#8499=ORIENTED_EDGE('',*,*,#5987,.T.);
#8500=ORIENTED_EDGE('',*,*,#5988,.T.);
#8501=ORIENTED_EDGE('',*,*,#5989,.T.);
#8502=ORIENTED_EDGE('',*,*,#5990,.T.);
#8503=ORIENTED_EDGE('',*,*,#5991,.T.);
#8504=ORIENTED_EDGE('',*,*,#5992,.T.);
#8505=ORIENTED_EDGE('',*,*,#5993,.T.);
#8506=ORIENTED_EDGE('',*,*,#5994,.T.);
#8507=ORIENTED_EDGE('',*,*,#5995,.T.);
#8508=ORIENTED_EDGE('',*,*,#5996,.T.);
#8509=ORIENTED_EDGE('',*,*,#5997,.T.);
#8510=ORIENTED_EDGE('',*,*,#5998,.T.);
#8511=ORIENTED_EDGE('',*,*,#5999,.T.);
#8512=ORIENTED_EDGE('',*,*,#6000,.T.);
#8513=ORIENTED_EDGE('',*,*,#6001,.F.);
#8514=ORIENTED_EDGE('',*,*,#5965,.T.);
#8515=ORIENTED_EDGE('',*,*,#6002,.T.);
#8516=ORIENTED_EDGE('',*,*,#6003,.T.);
#8517=ORIENTED_EDGE('',*,*,#5972,.F.);
#8518=ORIENTED_EDGE('',*,*,#5963,.T.);
#8519=ORIENTED_EDGE('',*,*,#6000,.F.);
#8520=ORIENTED_EDGE('',*,*,#6004,.T.);
#8521=ORIENTED_EDGE('',*,*,#6005,.T.);
#8522=ORIENTED_EDGE('',*,*,#6006,.F.);
#8523=ORIENTED_EDGE('',*,*,#6007,.T.);
#8524=ORIENTED_EDGE('',*,*,#6008,.F.);
#8525=ORIENTED_EDGE('',*,*,#5997,.F.);
#8526=ORIENTED_EDGE('',*,*,#6009,.F.);
#8527=ORIENTED_EDGE('',*,*,#6010,.F.);
#8528=ORIENTED_EDGE('',*,*,#6004,.F.);
#8529=ORIENTED_EDGE('',*,*,#5999,.F.);
#8530=ORIENTED_EDGE('',*,*,#6011,.T.);
#8531=ORIENTED_EDGE('',*,*,#6012,.T.);
#8532=ORIENTED_EDGE('',*,*,#5998,.F.);
#8533=ORIENTED_EDGE('',*,*,#6008,.T.);
#8534=ORIENTED_EDGE('',*,*,#6013,.T.);
#8535=ORIENTED_EDGE('',*,*,#6011,.F.);
#8536=ORIENTED_EDGE('',*,*,#6014,.F.);
#8537=ORIENTED_EDGE('',*,*,#6012,.F.);
#8538=ORIENTED_EDGE('',*,*,#6013,.F.);
#8539=ORIENTED_EDGE('',*,*,#6007,.F.);
#8540=ORIENTED_EDGE('',*,*,#6009,.T.);
#8541=ORIENTED_EDGE('',*,*,#5996,.F.);
#8542=ORIENTED_EDGE('',*,*,#6015,.T.);
#8543=ORIENTED_EDGE('',*,*,#6016,.T.);
#8544=ORIENTED_EDGE('',*,*,#6017,.F.);
#8545=ORIENTED_EDGE('',*,*,#6018,.T.);
#8546=ORIENTED_EDGE('',*,*,#6019,.F.);
#8547=ORIENTED_EDGE('',*,*,#5993,.F.);
#8548=ORIENTED_EDGE('',*,*,#6020,.F.);
#8549=ORIENTED_EDGE('',*,*,#6021,.F.);
#8550=ORIENTED_EDGE('',*,*,#6015,.F.);
#8551=ORIENTED_EDGE('',*,*,#5995,.F.);
#8552=ORIENTED_EDGE('',*,*,#6022,.T.);
#8553=ORIENTED_EDGE('',*,*,#6023,.T.);
#8554=ORIENTED_EDGE('',*,*,#5994,.F.);
#8555=ORIENTED_EDGE('',*,*,#6019,.T.);
#8556=ORIENTED_EDGE('',*,*,#6024,.T.);
#8557=ORIENTED_EDGE('',*,*,#6022,.F.);
#8558=ORIENTED_EDGE('',*,*,#6025,.F.);
#8559=ORIENTED_EDGE('',*,*,#6023,.F.);
#8560=ORIENTED_EDGE('',*,*,#6024,.F.);
#8561=ORIENTED_EDGE('',*,*,#6018,.F.);
#8562=ORIENTED_EDGE('',*,*,#6020,.T.);
#8563=ORIENTED_EDGE('',*,*,#5992,.F.);
#8564=ORIENTED_EDGE('',*,*,#6026,.T.);
#8565=ORIENTED_EDGE('',*,*,#6027,.T.);
#8566=ORIENTED_EDGE('',*,*,#6028,.F.);
#8567=ORIENTED_EDGE('',*,*,#6029,.T.);
#8568=ORIENTED_EDGE('',*,*,#6030,.F.);
#8569=ORIENTED_EDGE('',*,*,#5989,.F.);
#8570=ORIENTED_EDGE('',*,*,#6031,.F.);
#8571=ORIENTED_EDGE('',*,*,#6032,.F.);
#8572=ORIENTED_EDGE('',*,*,#6026,.F.);
#8573=ORIENTED_EDGE('',*,*,#5991,.F.);
#8574=ORIENTED_EDGE('',*,*,#6033,.T.);
#8575=ORIENTED_EDGE('',*,*,#6034,.T.);
#8576=ORIENTED_EDGE('',*,*,#5990,.F.);
#8577=ORIENTED_EDGE('',*,*,#6030,.T.);
#8578=ORIENTED_EDGE('',*,*,#6035,.T.);
#8579=ORIENTED_EDGE('',*,*,#6033,.F.);
#8580=ORIENTED_EDGE('',*,*,#6036,.F.);
#8581=ORIENTED_EDGE('',*,*,#6034,.F.);
#8582=ORIENTED_EDGE('',*,*,#6035,.F.);
#8583=ORIENTED_EDGE('',*,*,#6029,.F.);
#8584=ORIENTED_EDGE('',*,*,#6037,.F.);
#8585=ORIENTED_EDGE('',*,*,#6031,.T.);
#8586=ORIENTED_EDGE('',*,*,#5988,.F.);
#8587=ORIENTED_EDGE('',*,*,#6038,.T.);
#8588=ORIENTED_EDGE('',*,*,#6039,.T.);
#8589=ORIENTED_EDGE('',*,*,#6040,.F.);
#8590=ORIENTED_EDGE('',*,*,#6041,.T.);
#8591=ORIENTED_EDGE('',*,*,#6042,.F.);
#8592=ORIENTED_EDGE('',*,*,#5985,.F.);
#8593=ORIENTED_EDGE('',*,*,#6043,.F.);
#8594=ORIENTED_EDGE('',*,*,#6044,.F.);
#8595=ORIENTED_EDGE('',*,*,#6038,.F.);
#8596=ORIENTED_EDGE('',*,*,#5987,.F.);
#8597=ORIENTED_EDGE('',*,*,#6045,.T.);
#8598=ORIENTED_EDGE('',*,*,#6046,.T.);
#8599=ORIENTED_EDGE('',*,*,#5986,.F.);
#8600=ORIENTED_EDGE('',*,*,#6042,.T.);
#8601=ORIENTED_EDGE('',*,*,#6047,.T.);
#8602=ORIENTED_EDGE('',*,*,#6045,.F.);
#8603=ORIENTED_EDGE('',*,*,#6048,.F.);
#8604=ORIENTED_EDGE('',*,*,#6046,.F.);
#8605=ORIENTED_EDGE('',*,*,#6047,.F.);
#8606=ORIENTED_EDGE('',*,*,#6041,.F.);
#8607=ORIENTED_EDGE('',*,*,#6043,.T.);
#8608=ORIENTED_EDGE('',*,*,#5984,.F.);
#8609=ORIENTED_EDGE('',*,*,#6049,.T.);
#8610=ORIENTED_EDGE('',*,*,#6050,.T.);
#8611=ORIENTED_EDGE('',*,*,#6051,.F.);
#8612=ORIENTED_EDGE('',*,*,#6052,.T.);
#8613=ORIENTED_EDGE('',*,*,#6053,.F.);
#8614=ORIENTED_EDGE('',*,*,#5981,.F.);
#8615=ORIENTED_EDGE('',*,*,#6054,.F.);
#8616=ORIENTED_EDGE('',*,*,#6055,.F.);
#8617=ORIENTED_EDGE('',*,*,#6049,.F.);
#8618=ORIENTED_EDGE('',*,*,#5983,.F.);
#8619=ORIENTED_EDGE('',*,*,#6056,.T.);
#8620=ORIENTED_EDGE('',*,*,#6057,.T.);
#8621=ORIENTED_EDGE('',*,*,#5982,.F.);
#8622=ORIENTED_EDGE('',*,*,#6053,.T.);
#8623=ORIENTED_EDGE('',*,*,#6058,.T.);
#8624=ORIENTED_EDGE('',*,*,#6056,.F.);
#8625=ORIENTED_EDGE('',*,*,#6059,.F.);
#8626=ORIENTED_EDGE('',*,*,#6057,.F.);
#8627=ORIENTED_EDGE('',*,*,#6058,.F.);
#8628=ORIENTED_EDGE('',*,*,#6052,.F.);
#8629=ORIENTED_EDGE('',*,*,#6054,.T.);
#8630=ORIENTED_EDGE('',*,*,#5980,.F.);
#8631=ORIENTED_EDGE('',*,*,#6060,.T.);
#8632=ORIENTED_EDGE('',*,*,#6061,.T.);
#8633=ORIENTED_EDGE('',*,*,#6060,.F.);
#8634=ORIENTED_EDGE('',*,*,#5979,.F.);
#8635=ORIENTED_EDGE('',*,*,#6062,.T.);
#8636=ORIENTED_EDGE('',*,*,#6063,.T.);
#8637=ORIENTED_EDGE('',*,*,#6064,.F.);
#8638=ORIENTED_EDGE('',*,*,#6065,.F.);
#8639=ORIENTED_EDGE('',*,*,#6066,.F.);
#8640=ORIENTED_EDGE('',*,*,#6067,.T.);
#8641=ORIENTED_EDGE('',*,*,#6068,.F.);
#8642=ORIENTED_EDGE('',*,*,#5977,.F.);
#8643=ORIENTED_EDGE('',*,*,#5978,.F.);
#8644=ORIENTED_EDGE('',*,*,#6068,.T.);
#8645=ORIENTED_EDGE('',*,*,#6069,.T.);
#8646=ORIENTED_EDGE('',*,*,#6062,.F.);
#8647=ORIENTED_EDGE('',*,*,#6070,.F.);
#8648=ORIENTED_EDGE('',*,*,#6063,.F.);
#8649=ORIENTED_EDGE('',*,*,#6069,.F.);
#8650=ORIENTED_EDGE('',*,*,#6067,.F.);
#8651=ORIENTED_EDGE('',*,*,#6065,.T.);
#8652=ORIENTED_EDGE('',*,*,#5976,.F.);
#8653=ORIENTED_EDGE('',*,*,#6071,.T.);
#8654=ORIENTED_EDGE('',*,*,#6072,.T.);
#8655=ORIENTED_EDGE('',*,*,#6071,.F.);
#8656=ORIENTED_EDGE('',*,*,#5975,.F.);
#8657=ORIENTED_EDGE('',*,*,#6073,.T.);
#8658=ORIENTED_EDGE('',*,*,#6074,.T.);
#8659=ORIENTED_EDGE('',*,*,#6075,.F.);
#8660=ORIENTED_EDGE('',*,*,#6003,.F.);
#8661=ORIENTED_EDGE('',*,*,#6076,.F.);
#8662=ORIENTED_EDGE('',*,*,#6077,.T.);
#8663=ORIENTED_EDGE('',*,*,#6078,.F.);
#8664=ORIENTED_EDGE('',*,*,#5973,.F.);
#8665=ORIENTED_EDGE('',*,*,#5974,.F.);
#8666=ORIENTED_EDGE('',*,*,#6078,.T.);
#8667=ORIENTED_EDGE('',*,*,#6079,.T.);
#8668=ORIENTED_EDGE('',*,*,#6073,.F.);
#8669=ORIENTED_EDGE('',*,*,#6080,.F.);
#8670=ORIENTED_EDGE('',*,*,#6074,.F.);
#8671=ORIENTED_EDGE('',*,*,#6079,.F.);
#8672=ORIENTED_EDGE('',*,*,#6077,.F.);
#8673=ORIENTED_EDGE('',*,*,#6081,.F.);
#8674=ORIENTED_EDGE('',*,*,#6082,.T.);
#8675=ORIENTED_EDGE('',*,*,#6083,.T.);
#8676=ORIENTED_EDGE('',*,*,#6082,.F.);
#8677=ORIENTED_EDGE('',*,*,#6083,.F.);
#8678=ORIENTED_EDGE('',*,*,#6084,.F.);
#8679=ORIENTED_EDGE('',*,*,#6084,.T.);
#8680=ORIENTED_EDGE('',*,*,#6085,.T.);
#8681=ORIENTED_EDGE('',*,*,#6086,.T.);
#8682=ORIENTED_EDGE('',*,*,#6085,.F.);
#8683=ORIENTED_EDGE('',*,*,#6087,.F.);
#8684=ORIENTED_EDGE('',*,*,#6081,.T.);
#8685=ORIENTED_EDGE('',*,*,#6036,.T.);
#8686=ORIENTED_EDGE('',*,*,#6088,.T.);
#8687=ORIENTED_EDGE('',*,*,#6087,.T.);
#8688=ORIENTED_EDGE('',*,*,#6088,.F.);
#8689=ORIENTED_EDGE('',*,*,#6037,.T.);
#8690=ORIENTED_EDGE('',*,*,#6028,.T.);
#8691=ORIENTED_EDGE('',*,*,#6039,.F.);
#8692=ORIENTED_EDGE('',*,*,#6044,.T.);
#8693=ORIENTED_EDGE('',*,*,#6048,.T.);
#8694=ORIENTED_EDGE('',*,*,#6040,.T.);
#8695=ORIENTED_EDGE('',*,*,#6050,.F.);
#8696=ORIENTED_EDGE('',*,*,#6055,.T.);
#8697=ORIENTED_EDGE('',*,*,#6059,.T.);
#8698=ORIENTED_EDGE('',*,*,#6051,.T.);
#8699=ORIENTED_EDGE('',*,*,#6061,.F.);
#8700=ORIENTED_EDGE('',*,*,#6064,.T.);
#8701=ORIENTED_EDGE('',*,*,#6070,.T.);
#8702=ORIENTED_EDGE('',*,*,#6066,.T.);
#8703=ORIENTED_EDGE('',*,*,#6072,.F.);
#8704=ORIENTED_EDGE('',*,*,#6075,.T.);
#8705=ORIENTED_EDGE('',*,*,#6080,.T.);
#8706=ORIENTED_EDGE('',*,*,#6076,.T.);
#8707=ORIENTED_EDGE('',*,*,#6002,.F.);
#8708=ORIENTED_EDGE('',*,*,#5964,.T.);
#8709=ORIENTED_EDGE('',*,*,#5971,.T.);
#8710=ORIENTED_EDGE('',*,*,#5959,.T.);
#8711=ORIENTED_EDGE('',*,*,#6005,.F.);
#8712=ORIENTED_EDGE('',*,*,#6010,.T.);
#8713=ORIENTED_EDGE('',*,*,#6014,.T.);
#8714=ORIENTED_EDGE('',*,*,#6006,.T.);
#8715=ORIENTED_EDGE('',*,*,#6016,.F.);
#8716=ORIENTED_EDGE('',*,*,#6021,.T.);
#8717=ORIENTED_EDGE('',*,*,#6025,.T.);
#8718=ORIENTED_EDGE('',*,*,#6017,.T.);
#8719=ORIENTED_EDGE('',*,*,#6027,.F.);
#8720=ORIENTED_EDGE('',*,*,#6032,.T.);
#8721=ORIENTED_EDGE('',*,*,#6089,.F.);
#8722=ORIENTED_EDGE('',*,*,#6090,.T.);
#8723=ORIENTED_EDGE('',*,*,#6001,.T.);
#8724=ORIENTED_EDGE('',*,*,#6090,.F.);
#8725=ORIENTED_EDGE('',*,*,#6089,.T.);
#8726=ORIENTED_EDGE('',*,*,#6086,.F.);
#9709=ADVANCED_FACE('',(#2731),#1118,.F.);
#9710=ADVANCED_FACE('',(#2732),#1119,.F.);
#9711=ADVANCED_FACE('',(#2733),#1120,.F.);
#9712=ADVANCED_FACE('',(#2734),#1121,.F.);
#9713=ADVANCED_FACE('',(#2735,#455),#1122,.T.);
#9714=ADVANCED_FACE('',(#2736),#169,.T.);
#9715=ADVANCED_FACE('',(#2737),#170,.T.);
#9716=ADVANCED_FACE('',(#2738),#1123,.F.);
#9717=ADVANCED_FACE('',(#2739),#1124,.F.);
#9718=ADVANCED_FACE('',(#2740),#1125,.F.);
#9719=ADVANCED_FACE('',(#2741),#1126,.F.);
#9720=ADVANCED_FACE('',(#2742),#171,.T.);
#9721=ADVANCED_FACE('',(#2743),#1127,.F.);
#9722=ADVANCED_FACE('',(#2744),#1128,.F.);
#9723=ADVANCED_FACE('',(#2745),#1129,.F.);
#9724=ADVANCED_FACE('',(#2746),#1130,.F.);
#9725=ADVANCED_FACE('',(#2747),#172,.T.);
#9726=ADVANCED_FACE('',(#2748),#1131,.F.);
#9727=ADVANCED_FACE('',(#2749),#1132,.F.);
#9728=ADVANCED_FACE('',(#2750),#1133,.F.);
#9729=ADVANCED_FACE('',(#2751),#1134,.F.);
#9730=ADVANCED_FACE('',(#2752),#173,.T.);
#9731=ADVANCED_FACE('',(#2753),#1135,.F.);
#9732=ADVANCED_FACE('',(#2754),#1136,.F.);
#9733=ADVANCED_FACE('',(#2755),#1137,.F.);
#9734=ADVANCED_FACE('',(#2756),#1138,.F.);
#9735=ADVANCED_FACE('',(#2757),#174,.T.);
#9736=ADVANCED_FACE('',(#2758),#1139,.F.);
#9737=ADVANCED_FACE('',(#2759),#1140,.F.);
#9738=ADVANCED_FACE('',(#2760),#1141,.F.);
#9739=ADVANCED_FACE('',(#2761),#1142,.F.);
#9740=ADVANCED_FACE('',(#2762),#175,.T.);
#9741=ADVANCED_FACE('',(#2763),#1143,.F.);
#9742=ADVANCED_FACE('',(#2764),#1144,.F.);
#9743=ADVANCED_FACE('',(#2765),#1145,.F.);
#9744=ADVANCED_FACE('',(#2766),#1146,.F.);
#9745=ADVANCED_FACE('',(#2767),#176,.T.);
#9746=ADVANCED_FACE('',(#2768),#1147,.F.);
#9747=ADVANCED_FACE('',(#2769),#1148,.F.);
#9748=ADVANCED_FACE('',(#2770),#1149,.F.);
#9749=ADVANCED_FACE('',(#2771),#1150,.F.);
#9750=ADVANCED_FACE('',(#2772),#2344,.F.);
#9751=ADVANCED_FACE('',(#2773,#456),#1151,.F.);
#9752=ADVANCED_FACE('',(#2774),#2345,.F.);
#9753=ADVANCED_FACE('',(#2775,#457),#1152,.T.);
#9754=ADVANCED_FACE('',(#2776),#2346,.T.);
#9755=ADVANCED_FACE('',(#2777),#2347,.F.);
#9756=ADVANCED_FACE('',(#2778,#458),#1153,.T.);
#9889=CLOSED_SHELL('',(#9709,#9710,#9711,#9712,#9713,#9714,#9715,#9716,
#9717,#9718,#9719,#9720,#9721,#9722,#9723,#9724,#9725,#9726,#9727,#9728,
#9729,#9730,#9731,#9732,#9733,#9734,#9735,#9736,#9737,#9738,#9739,#9740,
#9741,#9742,#9743,#9744,#9745,#9746,#9747,#9748,#9749,#9750,#9751,#9752,
#9753,#9754,#9755,#9756));
#10598=AXIS2_PLACEMENT_3D('',#77387,#12299,#12300);
#10599=AXIS2_PLACEMENT_3D('',#77388,#12301,#12302);
#10600=AXIS2_PLACEMENT_3D('',#77401,#12307,#12308);
#10601=AXIS2_PLACEMENT_3D('',#77414,#12313,#12314);
#10602=AXIS2_PLACEMENT_3D('',#77417,#12317,#12318);
#10603=AXIS2_PLACEMENT_3D('',#77418,#12319,#12320);
#10604=AXIS2_PLACEMENT_3D('',#77419,#12321,#12322);
#10605=AXIS2_PLACEMENT_3D('',#77421,#12323,#12324);
#10606=AXIS2_PLACEMENT_3D('',#77429,#12328,#12329);
#10607=AXIS2_PLACEMENT_3D('',#77437,#12333,#12334);
#10608=AXIS2_PLACEMENT_3D('',#77445,#12338,#12339);
#10609=AXIS2_PLACEMENT_3D('',#77453,#12343,#12344);
#10610=AXIS2_PLACEMENT_3D('',#77461,#12348,#12349);
#10611=AXIS2_PLACEMENT_3D('',#77469,#12353,#12354);
#10612=AXIS2_PLACEMENT_3D('',#77476,#12358,#12359);
#10613=AXIS2_PLACEMENT_3D('',#77478,#12360,#12361);
#10614=AXIS2_PLACEMENT_3D('',#77479,#12362,#12363);
#10615=AXIS2_PLACEMENT_3D('',#77481,#12364,#12365);
#10616=AXIS2_PLACEMENT_3D('',#77485,#12366,#12367);
#10617=AXIS2_PLACEMENT_3D('',#77490,#12368,#12369);
#10618=AXIS2_PLACEMENT_3D('',#77491,#12370,#12371);
#10619=AXIS2_PLACEMENT_3D('',#77501,#12375,#12376);
#10620=AXIS2_PLACEMENT_3D('',#77507,#12380,#12381);
#10621=AXIS2_PLACEMENT_3D('',#77509,#12383,#12384);
#10622=AXIS2_PLACEMENT_3D('',#77510,#12385,#12386);
#10623=AXIS2_PLACEMENT_3D('',#77511,#12387,#12388);
#10624=AXIS2_PLACEMENT_3D('',#77516,#12389,#12390);
#10625=AXIS2_PLACEMENT_3D('',#77517,#12391,#12392);
#10626=AXIS2_PLACEMENT_3D('',#77527,#12396,#12397);
#10627=AXIS2_PLACEMENT_3D('',#77533,#12401,#12402);
#10628=AXIS2_PLACEMENT_3D('',#77535,#12404,#12405);
#10629=AXIS2_PLACEMENT_3D('',#77536,#12406,#12407);
#10630=AXIS2_PLACEMENT_3D('',#77537,#12408,#12409);
#10631=AXIS2_PLACEMENT_3D('',#77542,#12410,#12411);
#10632=AXIS2_PLACEMENT_3D('',#77543,#12412,#12413);
#10633=AXIS2_PLACEMENT_3D('',#77553,#12417,#12418);
#10634=AXIS2_PLACEMENT_3D('',#77559,#12422,#12423);
#10635=AXIS2_PLACEMENT_3D('',#77561,#12425,#12426);
#10636=AXIS2_PLACEMENT_3D('',#77563,#12427,#12428);
#10637=AXIS2_PLACEMENT_3D('',#77564,#12429,#12430);
#10638=AXIS2_PLACEMENT_3D('',#77565,#12431,#12432);
#10639=AXIS2_PLACEMENT_3D('',#77570,#12433,#12434);
#10640=AXIS2_PLACEMENT_3D('',#77571,#12435,#12436);
#10641=AXIS2_PLACEMENT_3D('',#77581,#12440,#12441);
#10642=AXIS2_PLACEMENT_3D('',#77587,#12445,#12446);
#10643=AXIS2_PLACEMENT_3D('',#77589,#12448,#12449);
#10644=AXIS2_PLACEMENT_3D('',#77590,#12450,#12451);
#10645=AXIS2_PLACEMENT_3D('',#77591,#12452,#12453);
#10646=AXIS2_PLACEMENT_3D('',#77596,#12454,#12455);
#10647=AXIS2_PLACEMENT_3D('',#77597,#12456,#12457);
#10648=AXIS2_PLACEMENT_3D('',#77607,#12461,#12462);
#10649=AXIS2_PLACEMENT_3D('',#77613,#12466,#12467);
#10650=AXIS2_PLACEMENT_3D('',#77615,#12469,#12470);
#10651=AXIS2_PLACEMENT_3D('',#77616,#12471,#12472);
#10652=AXIS2_PLACEMENT_3D('',#77617,#12473,#12474);
#10653=AXIS2_PLACEMENT_3D('',#77622,#12475,#12476);
#10654=AXIS2_PLACEMENT_3D('',#77623,#12477,#12478);
#10655=AXIS2_PLACEMENT_3D('',#77629,#12482,#12483);
#10656=AXIS2_PLACEMENT_3D('',#77639,#12487,#12488);
#10657=AXIS2_PLACEMENT_3D('',#77641,#12490,#12491);
#10658=AXIS2_PLACEMENT_3D('',#77642,#12492,#12493);
#10659=AXIS2_PLACEMENT_3D('',#77643,#12494,#12495);
#10660=AXIS2_PLACEMENT_3D('',#77648,#12496,#12497);
#10661=AXIS2_PLACEMENT_3D('',#77649,#12498,#12499);
#10662=AXIS2_PLACEMENT_3D('',#77655,#12503,#12504);
#10663=AXIS2_PLACEMENT_3D('',#77661,#12508,#12509);
#10664=AXIS2_PLACEMENT_3D('',#77663,#12511,#12512);
#10665=AXIS2_PLACEMENT_3D('',#77664,#12513,#12514);
#10666=AXIS2_PLACEMENT_3D('',#77665,#12515,#12516);
#10667=AXIS2_PLACEMENT_3D('',#77667,#12517,#12518);
#10668=AXIS2_PLACEMENT_3D('',#77670,#12520,#12521);
#10669=AXIS2_PLACEMENT_3D('',#77671,#12522,#12523);
#10670=AXIS2_PLACEMENT_3D('',#77673,#12524,#12525);
#10671=AXIS2_PLACEMENT_3D('',#77674,#12526,#12527);
#10672=AXIS2_PLACEMENT_3D('',#77677,#12529,#12530);
#10673=AXIS2_PLACEMENT_3D('',#77678,#12531,#12532);
#10674=AXIS2_PLACEMENT_3D('',#77680,#12533,#12534);
#10675=AXIS2_PLACEMENT_3D('',#77681,#12535,#12536);
#10676=AXIS2_PLACEMENT_3D('',#77683,#12538,#12539);
#10677=AXIS2_PLACEMENT_3D('',#77685,#12540,#12541);
#10678=AXIS2_PLACEMENT_3D('',#77687,#12543,#12544);
#12299=DIRECTION('axis',(0.,0.,1.));
#12300=DIRECTION('refdir',(1.,0.,0.));
#12301=DIRECTION('center_axis',(-0.707106781186548,-0.707106781186547,0.));
#12302=DIRECTION('ref_axis',(-0.707106781186547,0.707106781186548,0.));
#12303=DIRECTION('',(0.,0.,1.));
#12304=DIRECTION('',(-0.707106781186547,0.707106781186548,0.));
#12305=DIRECTION('',(0.,0.,-1.));
#12306=DIRECTION('',(-0.707106781186547,0.707106781186548,0.));
#12307=DIRECTION('center_axis',(0.707106781186548,0.707106781186547,0.));
#12308=DIRECTION('ref_axis',(0.707106781186547,-0.707106781186548,0.));
#12309=DIRECTION('',(0.,0.,-1.));
#12310=DIRECTION('',(0.707106781186547,-0.707106781186548,0.));
#12311=DIRECTION('',(0.,0.,-1.));
#12312=DIRECTION('',(0.707106781186547,-0.707106781186548,0.));
#12313=DIRECTION('center_axis',(-0.707106781186547,0.707106781186548,0.));
#12314=DIRECTION('ref_axis',(0.707106781186548,0.707106781186547,0.));
#12315=DIRECTION('',(0.707106781186548,0.707106781186547,0.));
#12316=DIRECTION('',(0.707106781186548,0.707106781186547,0.));
#12317=DIRECTION('center_axis',(0.,0.,-1.));
#12318=DIRECTION('ref_axis',(-0.707106781186547,0.707106781186548,0.));
#12319=DIRECTION('center_axis',(0.,0.,-1.));
#12320=DIRECTION('ref_axis',(1.,0.,0.));
#12321=DIRECTION('center_axis',(0.,0.,1.));
#12322=DIRECTION('ref_axis',(1.,0.,0.));
#12323=DIRECTION('center_axis',(0.,0.,1.));
#12324=DIRECTION('ref_axis',(1.,0.,0.));
#12325=DIRECTION('',(-1.,0.,0.));
#12326=DIRECTION('',(0.,1.,0.));
#12327=DIRECTION('',(1.,0.,0.));
#12328=DIRECTION('center_axis',(0.,0.,1.));
#12329=DIRECTION('ref_axis',(1.,0.,0.));
#12330=DIRECTION('',(-0.707106781186548,-0.707106781186548,0.));
#12331=DIRECTION('',(-0.707106781186548,0.707106781186548,0.));
#12332=DIRECTION('',(0.707106781186548,0.707106781186548,0.));
#12333=DIRECTION('center_axis',(0.,0.,1.));
#12334=DIRECTION('ref_axis',(1.,0.,0.));
#12335=DIRECTION('',(-6.12323399573677E-17,-1.,0.));
#12336=DIRECTION('',(-1.,6.12323399573677E-17,0.));
#12337=DIRECTION('',(6.12323399573677E-17,1.,0.));
#12338=DIRECTION('center_axis',(0.,0.,1.));
#12339=DIRECTION('ref_axis',(1.,0.,0.));
#12340=DIRECTION('',(0.707106781186547,-0.707106781186548,0.));
#12341=DIRECTION('',(-0.707106781186548,-0.707106781186547,0.));
#12342=DIRECTION('',(-0.707106781186547,0.707106781186548,0.));
#12343=DIRECTION('center_axis',(0.,0.,1.));
#12344=DIRECTION('ref_axis',(1.,0.,0.));
#12345=DIRECTION('',(1.,-1.22464679914735E-16,0.));
#12346=DIRECTION('',(-1.22464679914735E-16,-1.,0.));
#12347=DIRECTION('',(-1.,1.22464679914735E-16,0.));
#12348=DIRECTION('center_axis',(0.,0.,1.));
#12349=DIRECTION('ref_axis',(1.,0.,0.));
#12350=DIRECTION('',(0.707106781186548,0.707106781186547,0.));
#12351=DIRECTION('',(0.707106781186547,-0.707106781186548,0.));
#12352=DIRECTION('',(-0.707106781186548,-0.707106781186547,0.));
#12353=DIRECTION('center_axis',(0.,0.,1.));
#12354=DIRECTION('ref_axis',(1.,0.,0.));
#12355=DIRECTION('',(1.83697019872103E-16,1.,0.));
#12356=DIRECTION('',(1.,-1.83697019872103E-16,0.));
#12357=DIRECTION('',(-1.83697019872103E-16,-1.,0.));
#12358=DIRECTION('center_axis',(0.,0.,1.));
#12359=DIRECTION('ref_axis',(1.,0.,0.));
#12360=DIRECTION('center_axis',(0.,0.,1.));
#12361=DIRECTION('ref_axis',(1.,0.,0.));
#12362=DIRECTION('center_axis',(0.,0.,-1.));
#12363=DIRECTION('ref_axis',(1.,0.,0.));
#12364=DIRECTION('center_axis',(0.,0.,1.));
#12365=DIRECTION('ref_axis',(1.,0.,0.));
#12366=DIRECTION('center_axis',(0.,0.,-1.));
#12367=DIRECTION('ref_axis',(1.,0.,0.));
#12368=DIRECTION('center_axis',(0.,0.,1.));
#12369=DIRECTION('ref_axis',(1.,0.,0.));
#12370=DIRECTION('center_axis',(-1.,1.83697019872103E-16,0.));
#12371=DIRECTION('ref_axis',(1.83697019872103E-16,1.,0.));
#12372=DIRECTION('',(0.,0.,1.));
#12373=DIRECTION('',(1.83697019872103E-16,1.,0.));
#12374=DIRECTION('',(0.,0.,-1.));
#12375=DIRECTION('center_axis',(1.,-1.83697019872103E-16,0.));
#12376=DIRECTION('ref_axis',(-1.83697019872103E-16,-1.,0.));
#12377=DIRECTION('',(0.,0.,-1.));
#12378=DIRECTION('',(0.,0.,-1.));
#12379=DIRECTION('',(-1.83697019872103E-16,-1.,0.));
#12380=DIRECTION('center_axis',(1.83697019872103E-16,1.,0.));
#12381=DIRECTION('ref_axis',(1.,-1.83697019872103E-16,0.));
#12382=DIRECTION('',(1.,-1.83697019872103E-16,0.));
#12383=DIRECTION('center_axis',(0.,0.,-1.));
#12384=DIRECTION('ref_axis',(1.83697019872103E-16,1.,0.));
#12385=DIRECTION('center_axis',(0.,0.,-1.));
#12386=DIRECTION('ref_axis',(1.,0.,0.));
#12387=DIRECTION('center_axis',(0.,0.,-1.));
#12388=DIRECTION('ref_axis',(1.,0.,0.));
#12389=DIRECTION('center_axis',(0.,0.,1.));
#12390=DIRECTION('ref_axis',(1.,0.,0.));
#12391=DIRECTION('center_axis',(-0.707106781186547,0.707106781186548,0.));
#12392=DIRECTION('ref_axis',(0.707106781186548,0.707106781186547,0.));
#12393=DIRECTION('',(0.,0.,1.));
#12394=DIRECTION('',(0.707106781186548,0.707106781186547,0.));
#12395=DIRECTION('',(0.,0.,-1.));
#12396=DIRECTION('center_axis',(0.707106781186547,-0.707106781186548,0.));
#12397=DIRECTION('ref_axis',(-0.707106781186548,-0.707106781186547,0.));
#12398=DIRECTION('',(0.,0.,-1.));
#12399=DIRECTION('',(0.,0.,-1.));
#12400=DIRECTION('',(-0.707106781186548,-0.707106781186547,0.));
#12401=DIRECTION('center_axis',(0.707106781186548,0.707106781186547,0.));
#12402=DIRECTION('ref_axis',(0.707106781186547,-0.707106781186548,0.));
#12403=DIRECTION('',(0.707106781186547,-0.707106781186548,0.));
#12404=DIRECTION('center_axis',(0.,0.,-1.));
#12405=DIRECTION('ref_axis',(0.707106781186548,0.707106781186547,0.));
#12406=DIRECTION('center_axis',(0.,0.,-1.));
#12407=DIRECTION('ref_axis',(1.,0.,0.));
#12408=DIRECTION('center_axis',(0.,0.,-1.));
#12409=DIRECTION('ref_axis',(1.,0.,0.));
#12410=DIRECTION('center_axis',(0.,0.,1.));
#12411=DIRECTION('ref_axis',(1.,0.,0.));
#12412=DIRECTION('center_axis',(1.22464679914735E-16,1.,0.));
#12413=DIRECTION('ref_axis',(1.,-1.22464679914735E-16,0.));
#12414=DIRECTION('',(0.,0.,1.));
#12415=DIRECTION('',(1.,-1.22464679914735E-16,0.));
#12416=DIRECTION('',(0.,0.,-1.));
#12417=DIRECTION('center_axis',(-1.22464679914735E-16,-1.,0.));
#12418=DIRECTION('ref_axis',(-1.,1.22464679914735E-16,0.));
#12419=DIRECTION('',(0.,0.,-1.));
#12420=DIRECTION('',(0.,0.,-1.));
#12421=DIRECTION('',(-1.,1.22464679914735E-16,0.));
#12422=DIRECTION('center_axis',(1.,-1.22464679914735E-16,0.));
#12423=DIRECTION('ref_axis',(-1.22464679914735E-16,-1.,0.));
#12424=DIRECTION('',(-1.22464679914735E-16,-1.,0.));
#12425=DIRECTION('center_axis',(0.,0.,-1.));
#12426=DIRECTION('ref_axis',(1.,-1.22464679914735E-16,0.));
#12427=DIRECTION('center_axis',(0.,0.,-1.));
#12428=DIRECTION('ref_axis',(1.,0.,0.));
#12429=DIRECTION('center_axis',(0.,0.,-1.));
#12430=DIRECTION('ref_axis',(1.,0.,0.));
#12431=DIRECTION('center_axis',(0.,0.,-1.));
#12432=DIRECTION('ref_axis',(1.,0.,0.));
#12433=DIRECTION('center_axis',(0.,0.,1.));
#12434=DIRECTION('ref_axis',(1.,0.,0.));
#12435=DIRECTION('center_axis',(0.707106781186548,0.707106781186547,0.));
#12436=DIRECTION('ref_axis',(0.707106781186547,-0.707106781186548,0.));
#12437=DIRECTION('',(0.,0.,1.));
#12438=DIRECTION('',(0.707106781186547,-0.707106781186548,0.));
#12439=DIRECTION('',(0.,0.,-1.));
#12440=DIRECTION('center_axis',(-0.707106781186548,-0.707106781186547,0.));
#12441=DIRECTION('ref_axis',(-0.707106781186547,0.707106781186548,0.));
#12442=DIRECTION('',(0.,0.,-1.));
#12443=DIRECTION('',(0.,0.,-1.));
#12444=DIRECTION('',(-0.707106781186547,0.707106781186548,0.));
#12445=DIRECTION('center_axis',(0.707106781186547,-0.707106781186548,0.));
#12446=DIRECTION('ref_axis',(-0.707106781186548,-0.707106781186547,0.));
#12447=DIRECTION('',(-0.707106781186548,-0.707106781186547,0.));
#12448=DIRECTION('center_axis',(0.,0.,-1.));
#12449=DIRECTION('ref_axis',(0.707106781186547,-0.707106781186548,0.));
#12450=DIRECTION('center_axis',(0.,0.,-1.));
#12451=DIRECTION('ref_axis',(1.,0.,0.));
#12452=DIRECTION('center_axis',(0.,0.,-1.));
#12453=DIRECTION('ref_axis',(1.,0.,0.));
#12454=DIRECTION('center_axis',(0.,0.,1.));
#12455=DIRECTION('ref_axis',(1.,0.,0.));
#12456=DIRECTION('center_axis',(1.,-6.12323399573677E-17,0.));
#12457=DIRECTION('ref_axis',(-6.12323399573677E-17,-1.,0.));
#12458=DIRECTION('',(0.,0.,1.));
#12459=DIRECTION('',(-6.12323399573677E-17,-1.,0.));
#12460=DIRECTION('',(0.,0.,-1.));
#12461=DIRECTION('center_axis',(-1.,6.12323399573677E-17,0.));
#12462=DIRECTION('ref_axis',(6.12323399573677E-17,1.,0.));
#12463=DIRECTION('',(0.,0.,-1.));
#12464=DIRECTION('',(0.,0.,-1.));
#12465=DIRECTION('',(6.12323399573677E-17,1.,0.));
#12466=DIRECTION('center_axis',(-6.12323399573677E-17,-1.,0.));
#12467=DIRECTION('ref_axis',(-1.,6.12323399573677E-17,0.));
#12468=DIRECTION('',(-1.,6.12323399573677E-17,0.));
#12469=DIRECTION('center_axis',(0.,0.,-1.));
#12470=DIRECTION('ref_axis',(-6.12323399573677E-17,-1.,0.));
#12471=DIRECTION('center_axis',(0.,0.,-1.));
#12472=DIRECTION('ref_axis',(1.,0.,0.));
#12473=DIRECTION('center_axis',(0.,0.,-1.));
#12474=DIRECTION('ref_axis',(1.,0.,0.));
#12475=DIRECTION('center_axis',(0.,0.,1.));
#12476=DIRECTION('ref_axis',(1.,0.,0.));
#12477=DIRECTION('center_axis',(-0.707106781186548,0.707106781186548,0.));
#12478=DIRECTION('ref_axis',(0.707106781186548,0.707106781186548,0.));
#12479=DIRECTION('',(0.,0.,-1.));
#12480=DIRECTION('',(0.707106781186548,0.707106781186548,0.));
#12481=DIRECTION('',(0.,0.,-1.));
#12482=DIRECTION('center_axis',(0.707106781186548,-0.707106781186548,0.));
#12483=DIRECTION('ref_axis',(-0.707106781186548,-0.707106781186548,0.));
#12484=DIRECTION('',(0.,0.,1.));
#12485=DIRECTION('',(-0.707106781186548,-0.707106781186548,0.));
#12486=DIRECTION('',(0.,0.,-1.));
#12487=DIRECTION('center_axis',(-0.707106781186548,-0.707106781186548,0.));
#12488=DIRECTION('ref_axis',(-0.707106781186548,0.707106781186548,0.));
#12489=DIRECTION('',(-0.707106781186548,0.707106781186548,0.));
#12490=DIRECTION('center_axis',(0.,0.,-1.));
#12491=DIRECTION('ref_axis',(-0.707106781186548,-0.707106781186548,0.));
#12492=DIRECTION('center_axis',(0.,0.,-1.));
#12493=DIRECTION('ref_axis',(1.,0.,0.));
#12494=DIRECTION('center_axis',(0.,0.,-1.));
#12495=DIRECTION('ref_axis',(1.,0.,0.));
#12496=DIRECTION('center_axis',(0.,0.,1.));
#12497=DIRECTION('ref_axis',(1.,0.,0.));
#12498=DIRECTION('center_axis',(0.,1.,0.));
#12499=DIRECTION('ref_axis',(1.,0.,0.));
#12500=DIRECTION('',(0.,0.,-1.));
#12501=DIRECTION('',(1.,0.,0.));
#12502=DIRECTION('',(0.,0.,-1.));
#12503=DIRECTION('center_axis',(0.,-1.,0.));
#12504=DIRECTION('ref_axis',(-1.,0.,0.));
#12505=DIRECTION('',(0.,0.,1.));
#12506=DIRECTION('',(-1.,0.,0.));
#12507=DIRECTION('',(0.,0.,-1.));
#12508=DIRECTION('center_axis',(-1.,0.,0.));
#12509=DIRECTION('ref_axis',(0.,1.,0.));
#12510=DIRECTION('',(0.,1.,0.));
#12511=DIRECTION('center_axis',(0.,0.,-1.));
#12512=DIRECTION('ref_axis',(-1.,0.,0.));
#12513=DIRECTION('center_axis',(0.,0.,-1.));
#12514=DIRECTION('ref_axis',(1.,0.,0.));
#12515=DIRECTION('center_axis',(0.,0.,1.));
#12516=DIRECTION('ref_axis',(1.,0.,0.));
#12517=DIRECTION('center_axis',(0.,0.,1.));
#12518=DIRECTION('ref_axis',(1.,0.,0.));
#12519=DIRECTION('',(0.,0.,1.));
#12520=DIRECTION('center_axis',(0.,0.,1.));
#12521=DIRECTION('ref_axis',(1.,0.,0.));
#12522=DIRECTION('center_axis',(0.,0.,1.));
#12523=DIRECTION('ref_axis',(1.,0.,0.));
#12524=DIRECTION('center_axis',(0.,0.,-1.));
#12525=DIRECTION('ref_axis',(1.,0.,0.));
#12526=DIRECTION('center_axis',(0.,0.,1.));
#12527=DIRECTION('ref_axis',(1.,0.,0.));
#12528=DIRECTION('',(0.,0.,1.));
#12529=DIRECTION('center_axis',(0.,0.,1.));
#12530=DIRECTION('ref_axis',(1.,0.,0.));
#12531=DIRECTION('center_axis',(0.,0.,-1.));
#12532=DIRECTION('ref_axis',(-1.,0.,0.));
#12533=DIRECTION('center_axis',(0.,0.,1.));
#12534=DIRECTION('ref_axis',(1.,0.,0.));
#12535=DIRECTION('center_axis',(0.,0.,1.));
#12536=DIRECTION('ref_axis',(1.,0.,0.));
#12537=DIRECTION('',(0.,0.,-1.));
#12538=DIRECTION('center_axis',(0.,0.,1.));
#12539=DIRECTION('ref_axis',(1.,0.,0.));
#12540=DIRECTION('center_axis',(0.,0.,1.));
#12541=DIRECTION('ref_axis',(1.,0.,0.));
#12542=DIRECTION('',(0.,0.,1.));
#12543=DIRECTION('center_axis',(0.,0.,1.));
#12544=DIRECTION('ref_axis',(1.,0.,0.));
#77387=CARTESIAN_POINT('',(0.,0.,0.));
#77388=CARTESIAN_POINT('Origin',(0.989949493661167,0.897918471982869,13.75));
#77389=CARTESIAN_POINT('',(0.949277528782289,0.938590436861746,13.15));
#77390=CARTESIAN_POINT('',(0.949277528782289,0.938590436861746,13.6));
#77391=CARTESIAN_POINT('',(0.949277528782289,0.938590436861746,13.15));
#77392=CARTESIAN_POINT('',(0.82731493398826,1.06055303165577,13.15));
#77393=CARTESIAN_POINT('',(0.82731493398826,1.06055303165577,13.15));
#77394=CARTESIAN_POINT('',(0.82731493398826,1.06055303165577,13.75));
#77395=CARTESIAN_POINT('',(0.82731493398826,1.06055303165577,13.75));
#77396=CARTESIAN_POINT('',(0.906628408599113,0.981239557044922,13.75));
#77397=CARTESIAN_POINT('',(0.591941738241592,1.29592622740244,13.75));
#77398=CARTESIAN_POINT('Ctrl Pts',(0.94927752878229,0.938590436861745,13.6));
#77399=CARTESIAN_POINT('Ctrl Pts',(0.9275177734406,0.960350192203436,13.6765467245383));
#77400=CARTESIAN_POINT('Ctrl Pts',(0.906628408599113,0.981239557044923,
13.75));
#77401=CARTESIAN_POINT('Origin',(1.03944696834422,1.27268506601174,13.75));
#77402=CARTESIAN_POINT('',(1.16140956313825,1.15072247121771,13.6));
#77403=CARTESIAN_POINT('',(1.16140956313825,1.15072247121771,13.15));
#77404=CARTESIAN_POINT('',(1.16140956313825,1.15072247121771,13.15));
#77405=CARTESIAN_POINT('',(1.11876044295508,1.19337159140089,13.75));
#77406=CARTESIAN_POINT('Ctrl Pts',(1.11876044295508,1.19337159140089,13.75));
#77407=CARTESIAN_POINT('Ctrl Pts',(1.13964980776901,1.17248222658696,13.6765467246352));
#77408=CARTESIAN_POINT('Ctrl Pts',(1.16140956313825,1.15072247121771,13.6));
#77409=CARTESIAN_POINT('',(1.03944696834422,1.27268506601174,13.75));
#77410=CARTESIAN_POINT('',(0.722756492761103,1.58937554159486,13.75));
#77411=CARTESIAN_POINT('',(1.03944696834422,1.27268506601174,13.15));
#77412=CARTESIAN_POINT('',(1.03944696834422,1.27268506601174,13.75));
#77413=CARTESIAN_POINT('',(1.20208152801713,1.11005050633883,13.15));
#77414=CARTESIAN_POINT('Origin',(0.82731493398826,1.06055303165577,13.75));
#77415=CARTESIAN_POINT('',(1.03034794257725,1.26358604024477,13.75));
#77416=CARTESIAN_POINT('',(1.03944696834422,1.27268506601174,13.15));
#77417=CARTESIAN_POINT('Origin',(1.0146982310027,1.0853017689973,13.15));
#77418=CARTESIAN_POINT('Origin',(0.,2.1,13.15));
#77419=CARTESIAN_POINT('Origin',(0.6,2.1,13.75));
#77420=CARTESIAN_POINT('',(1.4321661914736,1.95,13.75));
#77421=CARTESIAN_POINT('Origin',(0.,2.1,13.75));
#77422=CARTESIAN_POINT('',(1.32,1.95,13.75));
#77423=CARTESIAN_POINT('',(1.075,1.95,13.75));
#77424=CARTESIAN_POINT('',(1.32,2.25,13.75));
#77425=CARTESIAN_POINT('',(1.32,2.025,13.75));
#77426=CARTESIAN_POINT('',(1.4321661914736,2.25,13.75));
#77427=CARTESIAN_POINT('',(0.96,2.25,13.75));
#77428=CARTESIAN_POINT('',(1.11876044295508,3.00662840859911,13.75));
#77429=CARTESIAN_POINT('Origin',(0.,2.1,13.75));
#77430=CARTESIAN_POINT('',(1.03944696834422,2.92731493398826,13.75));
#77431=CARTESIAN_POINT('',(0.804073772597556,2.69194173824159,13.75));
#77432=CARTESIAN_POINT('',(0.827314933988261,3.13944696834422,13.75));
#77433=CARTESIAN_POINT('',(1.13641395975523,2.83034794257725,13.75));
#77434=CARTESIAN_POINT('',(0.906628408599113,3.21876044295508,13.75));
#77435=CARTESIAN_POINT('',(0.510624458405139,2.8227564927611,13.75));
#77436=CARTESIAN_POINT('',(0.15,3.5321661914736,13.75));
#77437=CARTESIAN_POINT('Origin',(0.,2.1,13.75));
#77438=CARTESIAN_POINT('',(0.15,3.42,13.75));
#77439=CARTESIAN_POINT('',(0.15,2.875,13.75));
#77440=CARTESIAN_POINT('',(-0.15,3.42,13.75));
#77441=CARTESIAN_POINT('',(0.375,3.42,13.75));
#77442=CARTESIAN_POINT('',(-0.15,3.5321661914736,13.75));
#77443=CARTESIAN_POINT('',(-0.15,2.76,13.75));
#77444=CARTESIAN_POINT('',(-0.906628408599113,3.21876044295508,13.75));
#77445=CARTESIAN_POINT('Origin',(0.,2.1,13.75));
#77446=CARTESIAN_POINT('',(-0.82731493398826,3.13944696834423,13.75));
#77447=CARTESIAN_POINT('',(-0.291941738241592,2.60407377259756,13.75));
#77448=CARTESIAN_POINT('',(-1.03944696834422,2.92731493398826,13.75));
#77449=CARTESIAN_POINT('',(-0.730347942577251,3.23641395975523,13.75));
#77450=CARTESIAN_POINT('',(-1.11876044295508,3.00662840859911,13.75));
#77451=CARTESIAN_POINT('',(-0.422756492761103,2.31062445840514,13.75));
#77452=CARTESIAN_POINT('',(-1.4321661914736,2.25,13.75));
#77453=CARTESIAN_POINT('Origin',(0.,2.1,13.75));
#77454=CARTESIAN_POINT('',(-1.32,2.25,13.75));
#77455=CARTESIAN_POINT('',(-0.475,2.25,13.75));
#77456=CARTESIAN_POINT('',(-1.32,1.95,13.75));
#77457=CARTESIAN_POINT('',(-1.32,2.175,13.75));
#77458=CARTESIAN_POINT('',(-1.4321661914736,1.95,13.75));
#77459=CARTESIAN_POINT('',(-0.36,1.95,13.75));
#77460=CARTESIAN_POINT('',(-1.11876044295508,1.19337159140089,13.75));
#77461=CARTESIAN_POINT('Origin',(0.,2.1,13.75));
#77462=CARTESIAN_POINT('',(-1.03944696834423,1.27268506601174,13.75));
#77463=CARTESIAN_POINT('',(-0.504073772597556,1.80805826175841,13.75));
#77464=CARTESIAN_POINT('',(-0.827314933988261,1.06055303165578,13.75));
#77465=CARTESIAN_POINT('',(-0.836413959755234,1.06965205742275,13.75));
#77466=CARTESIAN_POINT('',(-0.906628408599113,0.981239557044923,13.75));
#77467=CARTESIAN_POINT('',(-0.210624458405139,1.6772435072389,13.75));
#77468=CARTESIAN_POINT('',(-0.15,0.667833808526399,13.75));
#77469=CARTESIAN_POINT('Origin',(0.,2.1,13.75));
#77470=CARTESIAN_POINT('',(-0.15,0.78,13.75));
#77471=CARTESIAN_POINT('',(-0.15,1.325,13.75));
#77472=CARTESIAN_POINT('',(0.149999999999999,0.78,13.75));
#77473=CARTESIAN_POINT('',(0.225,0.78,13.75));
#77474=CARTESIAN_POINT('',(0.149999999999999,0.667833808526399,13.75));
#77475=CARTESIAN_POINT('',(0.15,1.44,13.75));
#77476=CARTESIAN_POINT('Origin',(0.,2.1,13.75));
#77477=CARTESIAN_POINT('',(-0.6,2.1,13.75));
#77478=CARTESIAN_POINT('Origin',(0.,2.1,13.75));
#77479=CARTESIAN_POINT('Origin',(0.,2.1,13.675));
#77480=CARTESIAN_POINT('',(1.49248115565993,1.95,13.6));
#77481=CARTESIAN_POINT('Origin',(0.,2.1,13.6));
#77482=CARTESIAN_POINT('Ctrl Pts',(1.49248115565993,1.95,13.6));
#77483=CARTESIAN_POINT('Ctrl Pts',(1.46170821455344,1.95,13.6765467245093));
#77484=CARTESIAN_POINT('Ctrl Pts',(1.4321661914736,1.95,13.75));
#77485=CARTESIAN_POINT('Origin',(0.,2.1,13.675));
#77486=CARTESIAN_POINT('',(0.149999999999999,0.60751884434007,13.6));
#77487=CARTESIAN_POINT('Ctrl Pts',(0.149999999999999,0.667833808526398,
13.75));
#77488=CARTESIAN_POINT('Ctrl Pts',(0.149999999999999,0.638291785446644,
13.6765467245096));
#77489=CARTESIAN_POINT('Ctrl Pts',(0.149999999999999,0.607518844340069,
13.6));
#77490=CARTESIAN_POINT('Origin',(0.,2.1,13.6));
#77491=CARTESIAN_POINT('Origin',(-0.15,0.55,13.75));
#77492=CARTESIAN_POINT('',(-0.15,0.60751884434007,13.15));
#77493=CARTESIAN_POINT('',(-0.15,0.60751884434007,13.6));
#77494=CARTESIAN_POINT('',(-0.15,0.60751884434007,13.15));
#77495=CARTESIAN_POINT('',(-0.15,0.78,13.15));
#77496=CARTESIAN_POINT('',(-0.15,0.78,13.15));
#77497=CARTESIAN_POINT('',(-0.15,0.78,13.75));
#77498=CARTESIAN_POINT('Ctrl Pts',(-0.15,0.607518844340069,13.6));
#77499=CARTESIAN_POINT('Ctrl Pts',(-0.15,0.63829178544613,13.6765467245083));
#77500=CARTESIAN_POINT('Ctrl Pts',(-0.15,0.667833808526399,13.75));
#77501=CARTESIAN_POINT('Origin',(0.149999999999999,0.78,13.75));
#77502=CARTESIAN_POINT('',(0.149999999999999,0.60751884434007,13.15));
#77503=CARTESIAN_POINT('',(0.149999999999999,0.60751884434007,13.15));
#77504=CARTESIAN_POINT('',(0.149999999999999,0.78,13.15));
#77505=CARTESIAN_POINT('',(0.149999999999999,0.78,13.75));
#77506=CARTESIAN_POINT('',(0.149999999999999,0.55,13.15));
#77507=CARTESIAN_POINT('Origin',(-0.15,0.78,13.75));
#77508=CARTESIAN_POINT('',(0.149999999999999,0.78,13.15));
#77509=CARTESIAN_POINT('Origin',(-4.44089209850063E-16,0.665,13.15));
#77510=CARTESIAN_POINT('Origin',(0.,2.1,13.15));
#77511=CARTESIAN_POINT('Origin',(0.,2.1,13.675));
#77512=CARTESIAN_POINT('',(-0.94927752878229,0.938590436861747,13.6));
#77513=CARTESIAN_POINT('Ctrl Pts',(-0.906628408599113,0.981239557044923,
13.75));
#77514=CARTESIAN_POINT('Ctrl Pts',(-0.927517773496767,0.960350192147269,
13.6765467243408));
#77515=CARTESIAN_POINT('Ctrl Pts',(-0.94927752878229,0.938590436861746,
13.6));
#77516=CARTESIAN_POINT('Origin',(0.,2.1,13.6));
#77517=CARTESIAN_POINT('Origin',(-1.20208152801713,1.11005050633883,13.75));
#77518=CARTESIAN_POINT('',(-1.16140956313825,1.15072247121771,13.15));
#77519=CARTESIAN_POINT('',(-1.16140956313825,1.15072247121771,13.6));
#77520=CARTESIAN_POINT('',(-1.16140956313825,1.15072247121771,13.15));
#77521=CARTESIAN_POINT('',(-1.03944696834423,1.27268506601174,13.15));
#77522=CARTESIAN_POINT('',(-1.03944696834423,1.27268506601174,13.15));
#77523=CARTESIAN_POINT('',(-1.03944696834423,1.27268506601174,13.75));
#77524=CARTESIAN_POINT('Ctrl Pts',(-1.16140956313825,1.15072247121771,13.6));
#77525=CARTESIAN_POINT('Ctrl Pts',(-1.13964980779618,1.17248222655978,13.6765467245397));
#77526=CARTESIAN_POINT('Ctrl Pts',(-1.11876044295508,1.19337159140089,13.75));
#77527=CARTESIAN_POINT('Origin',(-0.827314933988261,1.06055303165578,13.75));
#77528=CARTESIAN_POINT('',(-0.94927752878229,0.938590436861747,13.15));
#77529=CARTESIAN_POINT('',(-0.94927752878229,0.938590436861747,13.15));
#77530=CARTESIAN_POINT('',(-0.827314933988261,1.06055303165578,13.15));
#77531=CARTESIAN_POINT('',(-0.827314933988261,1.06055303165578,13.75));
#77532=CARTESIAN_POINT('',(-0.989949493661167,0.897918471982869,13.15));
#77533=CARTESIAN_POINT('Origin',(-1.03944696834423,1.27268506601174,13.75));
#77534=CARTESIAN_POINT('',(-0.827314933988261,1.06055303165578,13.15));
#77535=CARTESIAN_POINT('Origin',(-1.0146982310027,1.0853017689973,13.15));
#77536=CARTESIAN_POINT('Origin',(0.,2.1,13.15));
#77537=CARTESIAN_POINT('Origin',(0.,2.1,13.675));
#77538=CARTESIAN_POINT('',(-1.49248115565993,1.95,13.6));
#77539=CARTESIAN_POINT('Ctrl Pts',(-1.4321661914736,1.95,13.75));
#77540=CARTESIAN_POINT('Ctrl Pts',(-1.46170821455336,1.95,13.6765467245096));
#77541=CARTESIAN_POINT('Ctrl Pts',(-1.49248115565993,1.95,13.6));
#77542=CARTESIAN_POINT('Origin',(0.,2.1,13.6));
#77543=CARTESIAN_POINT('Origin',(-1.55,2.25,13.75));
#77544=CARTESIAN_POINT('',(-1.49248115565993,2.25,13.15));
#77545=CARTESIAN_POINT('',(-1.49248115565993,2.25,13.6));
#77546=CARTESIAN_POINT('',(-1.49248115565993,2.25,13.15));
#77547=CARTESIAN_POINT('',(-1.32,2.25,13.15));
#77548=CARTESIAN_POINT('',(-1.32,2.25,13.15));
#77549=CARTESIAN_POINT('',(-1.32,2.25,13.75));
#77550=CARTESIAN_POINT('Ctrl Pts',(-1.49248115565993,2.25,13.6));
#77551=CARTESIAN_POINT('Ctrl Pts',(-1.46170821455336,2.25,13.6765467245096));
#77552=CARTESIAN_POINT('Ctrl Pts',(-1.4321661914736,2.25,13.75));
#77553=CARTESIAN_POINT('Origin',(-1.32,1.95,13.75));
#77554=CARTESIAN_POINT('',(-1.49248115565993,1.95,13.15));
#77555=CARTESIAN_POINT('',(-1.49248115565993,1.95,13.15));
#77556=CARTESIAN_POINT('',(-1.32,1.95,13.15));
#77557=CARTESIAN_POINT('',(-1.32,1.95,13.75));
#77558=CARTESIAN_POINT('',(-1.55,1.95,13.15));
#77559=CARTESIAN_POINT('Origin',(-1.32,2.25,13.75));
#77560=CARTESIAN_POINT('',(-1.32,1.95,13.15));
#77561=CARTESIAN_POINT('Origin',(-1.435,2.1,13.15));
#77562=CARTESIAN_POINT('',(-1.5,2.1,13.15));
#77563=CARTESIAN_POINT('Origin',(0.,2.1,13.15));
#77564=CARTESIAN_POINT('Origin',(0.,2.1,13.15));
#77565=CARTESIAN_POINT('Origin',(0.,2.1,13.675));
#77566=CARTESIAN_POINT('',(-1.16140956313825,3.04927752878229,13.6));
#77567=CARTESIAN_POINT('Ctrl Pts',(-1.11876044295508,3.00662840859911,13.75));
#77568=CARTESIAN_POINT('Ctrl Pts',(-1.13964980785287,3.02751777349691,13.6765467243403));
#77569=CARTESIAN_POINT('Ctrl Pts',(-1.16140956313825,3.04927752878229,13.6));
#77570=CARTESIAN_POINT('Origin',(0.,2.1,13.6));
#77571=CARTESIAN_POINT('Origin',(-0.989949493661166,3.30208152801713,13.75));
#77572=CARTESIAN_POINT('',(-0.949277528782289,3.26140956313825,13.15));
#77573=CARTESIAN_POINT('',(-0.949277528782289,3.26140956313825,13.6));
#77574=CARTESIAN_POINT('',(-0.949277528782289,3.26140956313825,13.15));
#77575=CARTESIAN_POINT('',(-0.82731493398826,3.13944696834423,13.15));
#77576=CARTESIAN_POINT('',(-0.82731493398826,3.13944696834423,13.15));
#77577=CARTESIAN_POINT('',(-0.82731493398826,3.13944696834423,13.75));
#77578=CARTESIAN_POINT('Ctrl Pts',(-0.94927752878229,3.26140956313825,13.6));
#77579=CARTESIAN_POINT('Ctrl Pts',(-0.927517773384816,3.23964980774078,
13.6765467247345));
#77580=CARTESIAN_POINT('Ctrl Pts',(-0.906628408599113,3.21876044295508,
13.75));
#77581=CARTESIAN_POINT('Origin',(-1.03944696834422,2.92731493398826,13.75));
#77582=CARTESIAN_POINT('',(-1.16140956313825,3.04927752878229,13.15));
#77583=CARTESIAN_POINT('',(-1.16140956313825,3.04927752878229,13.15));
#77584=CARTESIAN_POINT('',(-1.03944696834422,2.92731493398826,13.15));
#77585=CARTESIAN_POINT('',(-1.03944696834422,2.92731493398826,13.75));
#77586=CARTESIAN_POINT('',(-1.20208152801713,3.08994949366117,13.15));
#77587=CARTESIAN_POINT('Origin',(-0.82731493398826,3.13944696834423,13.75));
#77588=CARTESIAN_POINT('',(-1.03944696834422,2.92731493398826,13.15));
#77589=CARTESIAN_POINT('Origin',(-1.0146982310027,3.1146982310027,13.15));
#77590=CARTESIAN_POINT('Origin',(0.,2.1,13.15));
#77591=CARTESIAN_POINT('Origin',(0.,2.1,13.675));
#77592=CARTESIAN_POINT('',(-0.15,3.59248115565993,13.6));
#77593=CARTESIAN_POINT('Ctrl Pts',(-0.15,3.5321661914736,13.75));
#77594=CARTESIAN_POINT('Ctrl Pts',(-0.15,3.56170821455336,13.6765467245096));
#77595=CARTESIAN_POINT('Ctrl Pts',(-0.15,3.59248115565993,13.6));
#77596=CARTESIAN_POINT('Origin',(0.,2.1,13.6));
#77597=CARTESIAN_POINT('Origin',(0.15,3.65,13.75));
#77598=CARTESIAN_POINT('',(0.15,3.59248115565993,13.15));
#77599=CARTESIAN_POINT('',(0.15,3.59248115565993,13.6));
#77600=CARTESIAN_POINT('',(0.15,3.59248115565993,13.15));
#77601=CARTESIAN_POINT('',(0.15,3.42,13.15));
#77602=CARTESIAN_POINT('',(0.15,3.42,13.15));
#77603=CARTESIAN_POINT('',(0.15,3.42,13.75));
#77604=CARTESIAN_POINT('Ctrl Pts',(0.15,3.59248115565993,13.6));
#77605=CARTESIAN_POINT('Ctrl Pts',(0.15,3.56170821455336,13.6765467245096));
#77606=CARTESIAN_POINT('Ctrl Pts',(0.15,3.5321661914736,13.75));
#77607=CARTESIAN_POINT('Origin',(-0.15,3.42,13.75));
#77608=CARTESIAN_POINT('',(-0.15,3.59248115565993,13.15));
#77609=CARTESIAN_POINT('',(-0.15,3.59248115565993,13.15));
#77610=CARTESIAN_POINT('',(-0.15,3.42,13.15));
#77611=CARTESIAN_POINT('',(-0.15,3.42,13.75));
#77612=CARTESIAN_POINT('',(-0.15,3.65,13.15));
#77613=CARTESIAN_POINT('Origin',(0.15,3.42,13.75));
#77614=CARTESIAN_POINT('',(-0.15,3.42,13.15));
#77615=CARTESIAN_POINT('Origin',(0.,3.535,13.15));
#77616=CARTESIAN_POINT('Origin',(0.,2.1,13.15));
#77617=CARTESIAN_POINT('Origin',(0.,2.1,13.675));
#77618=CARTESIAN_POINT('',(0.94927752878229,3.26140956313825,13.6));
#77619=CARTESIAN_POINT('Ctrl Pts',(0.906628408599113,3.21876044295508,13.75));
#77620=CARTESIAN_POINT('Ctrl Pts',(0.92751777344062,3.23964980779658,13.6765467245382));
#77621=CARTESIAN_POINT('Ctrl Pts',(0.94927752878229,3.26140956313825,13.6));
#77622=CARTESIAN_POINT('Origin',(0.,2.1,13.6));
#77623=CARTESIAN_POINT('Origin',(0.827314933988261,3.13944696834422,13.75));
#77624=CARTESIAN_POINT('',(0.827314933988261,3.13944696834422,13.15));
#77625=CARTESIAN_POINT('',(0.827314933988261,3.13944696834422,13.75));
#77626=CARTESIAN_POINT('',(0.94927752878229,3.26140956313825,13.15));
#77627=CARTESIAN_POINT('',(0.989949493661167,3.30208152801713,13.15));
#77628=CARTESIAN_POINT('',(0.94927752878229,3.26140956313825,13.15));
#77629=CARTESIAN_POINT('Origin',(1.20208152801713,3.08994949366117,13.75));
#77630=CARTESIAN_POINT('',(1.16140956313825,3.04927752878229,13.6));
#77631=CARTESIAN_POINT('Ctrl Pts',(1.16140956313825,3.04927752878229,13.6));
#77632=CARTESIAN_POINT('Ctrl Pts',(1.13964980779658,3.02751777344062,13.6765467245382));
#77633=CARTESIAN_POINT('Ctrl Pts',(1.11876044295508,3.00662840859911,13.75));
#77634=CARTESIAN_POINT('',(1.16140956313825,3.04927752878229,13.15));
#77635=CARTESIAN_POINT('',(1.16140956313825,3.04927752878229,13.15));
#77636=CARTESIAN_POINT('',(1.03944696834422,2.92731493398826,13.15));
#77637=CARTESIAN_POINT('',(1.03944696834422,2.92731493398826,13.15));
#77638=CARTESIAN_POINT('',(1.03944696834422,2.92731493398826,13.75));
#77639=CARTESIAN_POINT('Origin',(1.03944696834422,2.92731493398826,13.75));
#77640=CARTESIAN_POINT('',(0.827314933988261,3.13944696834422,13.15));
#77641=CARTESIAN_POINT('Origin',(1.0146982310027,3.1146982310027,13.15));
#77642=CARTESIAN_POINT('Origin',(0.,2.1,13.15));
#77643=CARTESIAN_POINT('Origin',(0.,2.1,13.675));
#77644=CARTESIAN_POINT('',(1.49248115565993,2.25,13.6));
#77645=CARTESIAN_POINT('Ctrl Pts',(1.4321661914736,2.25,13.75));
#77646=CARTESIAN_POINT('Ctrl Pts',(1.46170821455344,2.25,13.6765467245093));
#77647=CARTESIAN_POINT('Ctrl Pts',(1.49248115565993,2.25,13.6));
#77648=CARTESIAN_POINT('Origin',(0.,2.1,13.6));
#77649=CARTESIAN_POINT('Origin',(1.32,2.25,13.75));
#77650=CARTESIAN_POINT('',(1.32,2.25,13.15));
#77651=CARTESIAN_POINT('',(1.32,2.25,13.75));
#77652=CARTESIAN_POINT('',(1.49248115565993,2.25,13.15));
#77653=CARTESIAN_POINT('',(1.55,2.25,13.15));
#77654=CARTESIAN_POINT('',(1.49248115565993,2.25,13.15));
#77655=CARTESIAN_POINT('Origin',(1.55,1.95,13.75));
#77656=CARTESIAN_POINT('',(1.49248115565993,1.95,13.15));
#77657=CARTESIAN_POINT('',(1.49248115565993,1.95,13.15));
#77658=CARTESIAN_POINT('',(1.32,1.95,13.15));
#77659=CARTESIAN_POINT('',(1.32,1.95,13.15));
#77660=CARTESIAN_POINT('',(1.32,1.95,13.75));
#77661=CARTESIAN_POINT('Origin',(1.32,1.95,13.75));
#77662=CARTESIAN_POINT('',(1.32,2.25,13.15));
#77663=CARTESIAN_POINT('Origin',(1.435,2.1,13.15));
#77664=CARTESIAN_POINT('Origin',(0.,2.1,13.15));
#77665=CARTESIAN_POINT('Origin',(0.,2.1,13.035));
#77666=CARTESIAN_POINT('',(-1.1,2.1,12.7));
#77667=CARTESIAN_POINT('Origin',(0.,2.1,12.7));
#77668=CARTESIAN_POINT('',(-1.1,2.1,13.42));
#77669=CARTESIAN_POINT('',(-1.1,2.1,13.035));
#77670=CARTESIAN_POINT('Origin',(0.,2.1,13.42));
#77671=CARTESIAN_POINT('Origin',(0.,2.1,13.42));
#77672=CARTESIAN_POINT('',(-0.46,2.1,13.42));
#77673=CARTESIAN_POINT('Origin',(0.,2.1,13.42));
#77674=CARTESIAN_POINT('Origin',(0.,2.1,13.1));
#77675=CARTESIAN_POINT('',(-0.46,2.1,13.5));
#77676=CARTESIAN_POINT('',(-0.46,2.1,13.1));
#77677=CARTESIAN_POINT('Origin',(0.,2.1,13.5));
#77678=CARTESIAN_POINT('Origin',(1.5,2.1,12.7));
#77679=CARTESIAN_POINT('',(-1.5,2.1,12.7));
#77680=CARTESIAN_POINT('Origin',(0.,2.1,12.7));
#77681=CARTESIAN_POINT('Origin',(0.,2.1,13.15));
#77682=CARTESIAN_POINT('',(-1.5,2.1,13.15));
#77683=CARTESIAN_POINT('Origin',(0.,2.1,13.625));
#77684=CARTESIAN_POINT('',(-0.6,2.1,13.5));
#77685=CARTESIAN_POINT('Origin',(0.,2.1,13.5));
#77686=CARTESIAN_POINT('',(-0.6,2.1,13.625));
#77687=CARTESIAN_POINT('Origin',(0.46,2.1,13.5));
#85759=UNCERTAINTY_MEASURE_WITH_UNIT(LENGTH_MEASURE(0.001),#85790,
'DISTANCE_ACCURACY_VALUE',
'Maximum model space distance between geometric entities at asserted c
onnectivities');
#85769=UNCERTAINTY_MEASURE_WITH_UNIT(LENGTH_MEASURE(0.001),#85790,
'DISTANCE_ACCURACY_VALUE',
'Maximum model space distance between geometric entities at asserted c
onnectivities');
#85779=(
GEOMETRIC_REPRESENTATION_CONTEXT(3)
GLOBAL_UNCERTAINTY_ASSIGNED_CONTEXT((#85759))
GLOBAL_UNIT_ASSIGNED_CONTEXT((#85790,#85792,#85793))
REPRESENTATION_CONTEXT('','3D')
);
#85789=(
GEOMETRIC_REPRESENTATION_CONTEXT(3)
GLOBAL_UNCERTAINTY_ASSIGNED_CONTEXT((#85769))
GLOBAL_UNIT_ASSIGNED_CONTEXT((#85790,#85792,#85793))
REPRESENTATION_CONTEXT('','3D')
);
#85790=(
LENGTH_UNIT()
NAMED_UNIT(*)
SI_UNIT(.CENTI.,.METRE.)
);
#85792=(
NAMED_UNIT(*)
PLANE_ANGLE_UNIT()
SI_UNIT($,.RADIAN.)
);
#85793=(
NAMED_UNIT(*)
SI_UNIT($,.STERADIAN.)
SOLID_ANGLE_UNIT()
);
#85803=SHAPE_DEFINITION_REPRESENTATION(#85822,#85871);
#85822=PRODUCT_DEFINITION_SHAPE('',$,#85891);
#85871=SHAPE_REPRESENTATION('',(#10598),#85779);
#85881=PRODUCT_DEFINITION_CONTEXT('part definition',#85940,'design');
#85891=PRODUCT_DEFINITION('Spindle Bearing Cap','Spindle Bearing Cap',#85910,
#85881);
#85910=PRODUCT_DEFINITION_FORMATION('',$,#85951);
#85940=APPLICATION_CONTEXT(
'Core Data for Automotive Mechanical Design Process');
#85941=PRODUCT_CONTEXT('part definition',#85940,'mechanical');
#85951=PRODUCT('Spindle Bearing Cap','Spindle Bearing Cap',$,(#85941));
#85970=PRESENTATION_STYLE_ASSIGNMENT((#85988));
#85988=SURFACE_STYLE_USAGE(.BOTH.,#86006);
#86006=SURFACE_SIDE_STYLE('',(#86024));
#86024=SURFACE_STYLE_FILL_AREA(#86042);
#86042=FILL_AREA_STYLE('Opaque(30,30,33)',(#86060));
#86060=FILL_AREA_STYLE_COLOUR('Opaque(30,30,33)',#86078);
#86078=COLOUR_RGB('Opaque(30,30,33)', 0.40784314, 0.44705882, 0.49803922);
ENDSEC;
END-ISO-10303-21;
